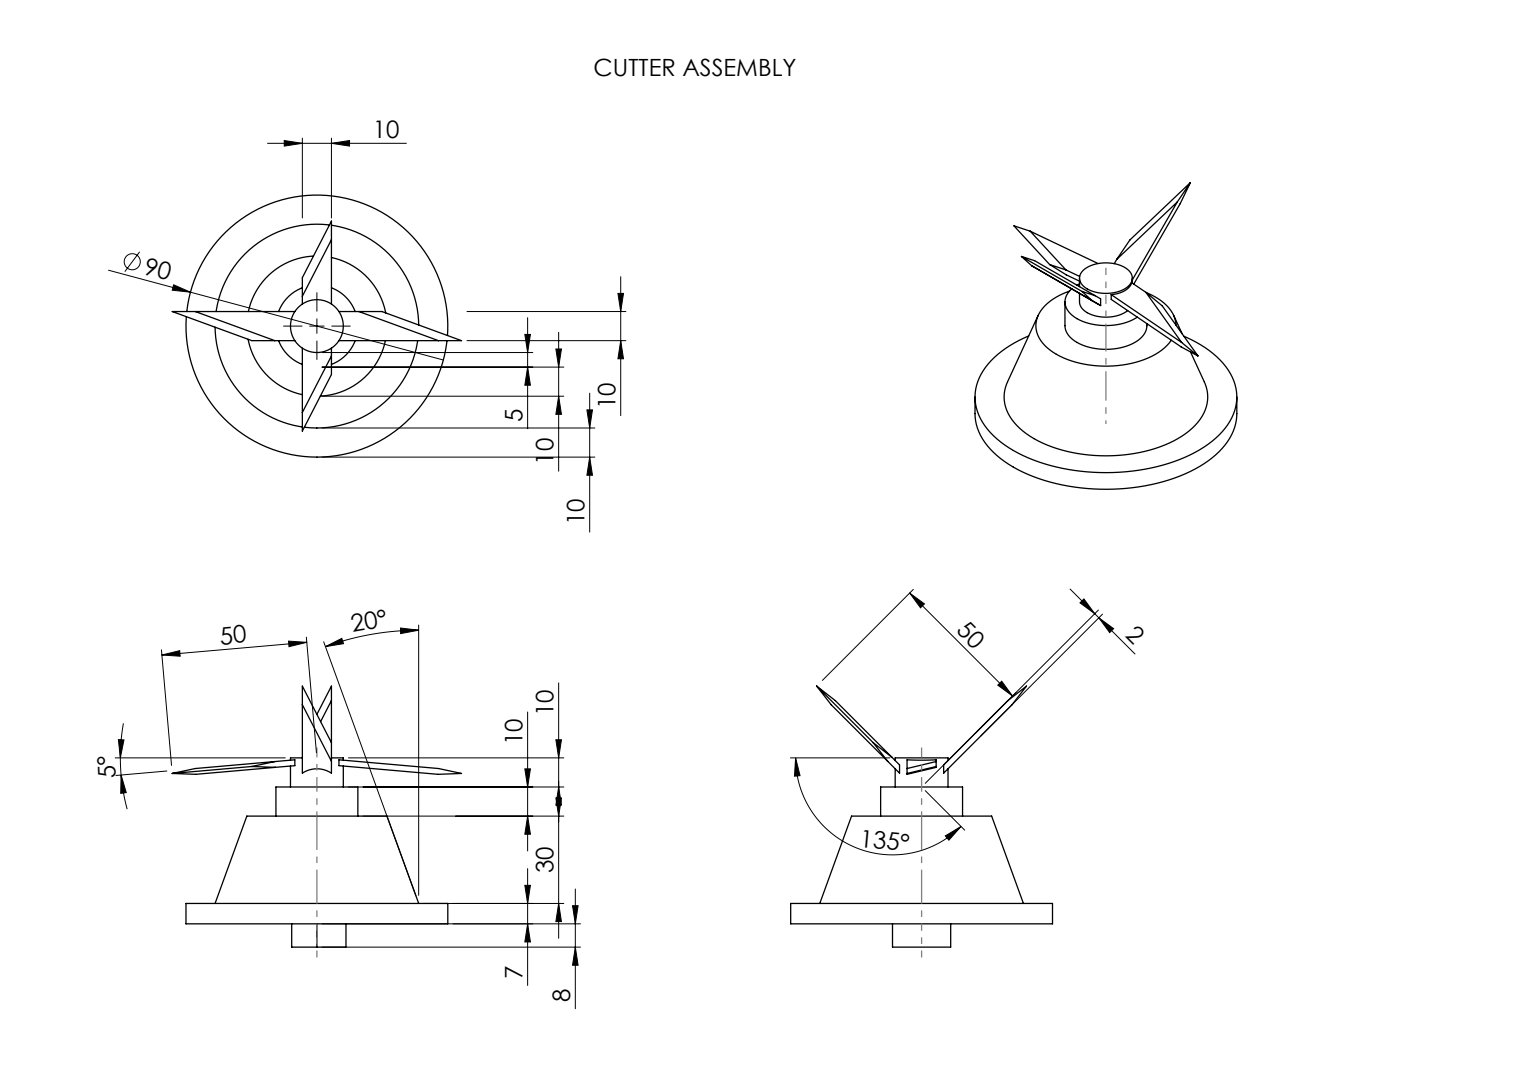
ISO-10303-21;
HEADER;
FILE_DESCRIPTION (('STEP AP214'),
    '1' );
FILE_NAME ('cutter assembly.step',
    '2026-10-09T15:02:13',
    ( '' ),
    ( '' ),
    'SwSTEP 2.0',
    'SolidWorks 2026',
    '' );
FILE_SCHEMA (( 'AUTOMOTIVE_DESIGN' ));
ENDSEC;

DATA;
#1=EDGE_CURVE ( 'NONE', #9758, #2312, #3659, .T. ) ;
#30=LINE ( 'NONE', #10110, #8655 ) ;
#58=VERTEX_POINT ( 'NONE', #12787 ) ;
#66=CARTESIAN_POINT ( 'NONE',  ( 9.262651381018932677E-15, 92.00000000000001421, -9.080892972013931086 ) ) ;
#71=ADVANCED_FACE ( 'NONE', ( #2644 ), #15361, .T. ) ;
#93=AXIS2_PLACEMENT_3D ( 'NONE', #810, #7225, #14526 ) ;
#117=CARTESIAN_POINT ( 'NONE',  ( -3.505380114644273348, 97.73782665365220623, 8.566253778398339236 ) ) ;
#119=ORIENTED_EDGE ( 'NONE', *, *, #8529, .T. ) ;
#143=CARTESIAN_POINT ( 'NONE',  ( 5.000000000000000000, 90.58578643762692195, -1.414213562373097588 ) ) ;
#172=VERTEX_POINT ( 'NONE', #11782 ) ;
#182=CARTESIAN_POINT ( 'NONE',  ( 9.227956911499398113E-15, 102.0000000000000142, -9.080892972013931086 ) ) ;
#202=CARTESIAN_POINT ( 'NONE',  ( 5.000000000000000000, 96.75198296766784267, -7.580410092414001433 ) ) ;
#213=EDGE_CURVE ( 'NONE', #982, #10751, #1081, .T. ) ;
#214=DIRECTION ( 'NONE',  ( 6.938893903907231459E-18, -1.000000000000000000, -5.551115123125782702E-17 ) ) ;
#218=PLANE ( 'NONE',  #7160 ) ;
#231=CARTESIAN_POINT ( 'NONE',  ( -49.72257916183962578, 96.64601816452537264, -5.000000000000008882 ) ) ;
#235=CARTESIAN_POINT ( 'NONE',  ( 9.332040320058006538E-15, 82.00000000000001421, -14.08089297201393286 ) ) ;
#296=DIRECTION ( 'NONE',  ( 0.000000000000000000, -0.7071067811865487940, -0.7071067811865463515 ) ) ;
#306=VERTEX_POINT ( 'NONE', #6172 ) ;
#321=CARTESIAN_POINT ( 'NONE',  ( -0.1743114854953159432, 100.0076106038165165, -5.000000000000000000 ) ) ;
#332=VERTEX_POINT ( 'NONE', #9993 ) ;
#335=DIRECTION ( 'NONE',  ( -5.069245582283711292E-17, -1.000000000000000000, 8.780190904559502465E-17 ) ) ;
#357=CARTESIAN_POINT ( 'NONE',  ( 5.000000000000000000, 102.0000000000000142, -7.580410092414002321 ) ) ;
#401=COLOUR_RGB ( '', 0.72549020, 0.75294118, 0.79215686) ;
#416=DIRECTION ( 'NONE',  ( -0.3420201433256697121, -0.6644630243886754384, 0.6644630243886734400 ) ) ;
#431=VECTOR ( 'NONE', #921, 1000.000000000000114 ) ;
#437=CARTESIAN_POINT ( 'NONE',  ( 9.234334497652928468E-15, 101.0808929720139702, -9.080892972013931086 ) ) ;
#456=CARTESIAN_POINT ( 'NONE',  ( -7.580410092413954359, 101.3368000520362813, 5.000000000000000000 ) ) ;
#457=CARTESIAN_POINT ( 'NONE',  ( 9.574901606694759531E-15, 52.00000000000001421, -2.191293403013901479E-14 ) ) ;
#460=ADVANCED_FACE ( 'NONE', ( #10847 ), #14901, .F. ) ;
#467=ORIENTED_EDGE ( 'NONE', *, *, #5813, .T. ) ;
#473=CARTESIAN_POINT ( 'NONE',  ( 5.000000000000000000, 92.00000000000001421, 0.000000000000000000 ) ) ;
#477=DIRECTION ( 'NONE',  ( 0.9361168066628590134, -0.08189960831908912886, 0.3420201433256691570 ) ) ;
#481=FILL_AREA_STYLE_COLOUR ( '', #401 ) ;
#487=ORIENTED_EDGE ( 'NONE', *, *, #6442, .T. ) ;
#492=AXIS2_PLACEMENT_3D ( 'NONE', #10068, #2407, #11397 ) ;
#499=FACE_OUTER_BOUND ( 'NONE', #6302, .T. ) ;
#506=ADVANCED_FACE ( 'NONE', ( #2101 ), #15988, .T. ) ;
#507=FACE_OUTER_BOUND ( 'NONE', #6954, .T. ) ;
#529=ADVANCED_FACE ( 'NONE', ( #2178 ), #12250, .T. ) ;
#536=DIRECTION ( 'NONE',  ( 0.000000000000000000, -1.541976423090494894E-16, -1.000000000000000000 ) ) ;
#537=DIRECTION ( 'NONE',  ( -0.000000000000000000, -0.6143407043256620126, -0.7890408728378077718 ) ) ;
#545=ORIENTED_EDGE ( 'NONE', *, *, #14628, .F. ) ;
#548=ORIENTED_EDGE ( 'NONE', *, *, #4265, .T. ) ;
#558=CARTESIAN_POINT ( 'NONE',  ( 1.875620865444973696E-15, 37.00000000000001421, -3.248670634687016947E-15 ) ) ;
#600=AXIS2_PLACEMENT_3D ( 'NONE', #14454, #6924, #1670 ) ;
#606=EDGE_CURVE ( 'NONE', #16014, #2610, #15398, .T. ) ;
#622=EDGE_LOOP ( 'NONE', ( #7600, #10634, #1804, #893 ) ) ;
#624=ORIENTED_EDGE ( 'NONE', *, *, #14015, .F. ) ;
#642=( GEOMETRIC_REPRESENTATION_CONTEXT ( 3 ) GLOBAL_UNCERTAINTY_ASSIGNED_CONTEXT ( ( #2937 ) ) GLOBAL_UNIT_ASSIGNED_CONTEXT ( ( #15209, #12566, #3759 ) ) REPRESENTATION_CONTEXT ( 'NONE', 'WORKASPACE' ) );
#648=DIRECTION ( 'NONE',  ( 0.000000000000000000, 8.780190904559502465E-17, 1.000000000000000000 ) ) ;
#650=ORIENTED_EDGE ( 'NONE', *, *, #1309, .F. ) ;
#660=DIRECTION ( 'NONE',  ( 0.000000000000000000, 0.000000000000000000, 1.000000000000000000 ) ) ;
#664=DIRECTION ( 'NONE',  ( -0.9961946980917455452, 0.08715574274765797158, 0.000000000000000000 ) ) ;
#668=AXIS2_PLACEMENT_3D ( 'NONE', #6556, #5317, #14175 ) ;
#677=VECTOR ( 'NONE', #999, 1000.000000000000114 ) ;
#686=CARTESIAN_POINT ( 'NONE',  ( 5.000000000000000000, 92.00000000000001421, 0.000000000000000000 ) ) ;
#698=AXIS2_PLACEMENT_3D ( 'NONE', #9570, #3238, #12296 ) ;
#700=ORIENTED_EDGE ( 'NONE', *, *, #4864, .F. ) ;
#706=VECTOR ( 'NONE', #3589, 1000.000000000000114 ) ;
#733=CIRCLE ( 'NONE', #6335, 9.080892972013911546 ) ;
#757=VECTOR ( 'NONE', #2822, 1000.000000000000000 ) ;
#759=DIRECTION ( 'NONE',  ( 0.9361168066628589024, 0.08189960831908940642, 0.3420201433256691570 ) ) ;
#784=CARTESIAN_POINT ( 'NONE',  ( 9.642970592016636644, 101.1563493904846780, 1.872989114519530984 ) ) ;
#798=VERTEX_POINT ( 'NONE', #9337 ) ;
#810=CARTESIAN_POINT ( 'NONE',  ( 9.297345850538470396E-15, 92.00000000000001421, -1.969248798088869855E-14 ) ) ;
#815=EDGE_CURVE ( 'NONE', #11124, #14188, #16130, .T. ) ;
#840=ORIENTED_EDGE ( 'NONE', *, *, #2746, .T. ) ;
#853=DIRECTION ( 'NONE',  ( 0.000000000000000000, 0.7071067811865487940, 0.7071067811865463515 ) ) ;
#877=ORIENTED_EDGE ( 'NONE', *, *, #7745, .T. ) ;
#893=ORIENTED_EDGE ( 'NONE', *, *, #4265, .F. ) ;
#894=VERTEX_POINT ( 'NONE', #14312 ) ;
#899=DIRECTION ( 'NONE',  ( -1.000000000000000000, 0.000000000000000000, -0.000000000000000000 ) ) ;
#907=ADVANCED_FACE ( 'NONE', ( #507 ), #6097, .T. ) ;
#916=ADVANCED_FACE ( 'NONE', ( #11164 ), #4772, .F. ) ;
#921=DIRECTION ( 'NONE',  ( 0.9361168066628589024, 0.08189960831908940642, 0.3420201433256691015 ) ) ;
#948=CARTESIAN_POINT ( 'NONE',  ( 7.580410092413973011, 101.3368000520362813, 5.000000000000000000 ) ) ;
#953=AXIS2_PLACEMENT_3D ( 'NONE', #5436, #10499, #15557 ) ;
#962=ORIENTED_EDGE ( 'NONE', *, *, #15661, .F. ) ;
#965=CARTESIAN_POINT ( 'NONE',  ( 9.297345850538470396E-15, 92.00000000000001421, -1.969248798088869855E-14 ) ) ;
#982=VERTEX_POINT ( 'NONE', #15894 ) ;
#991=DIRECTION ( 'NONE',  ( -0.9961946980917455452, -0.08715574274765824914, 0.000000000000000000 ) ) ;
#999=DIRECTION ( 'NONE',  ( 0.9961946980917455452, 0.08715574274765823526, -0.000000000000000000 ) ) ;
#1008=DIRECTION ( 'NONE',  ( 0.000000000000000000, -5.551115123125782702E-17, 1.000000000000000000 ) ) ;
#1023=ORIENTED_EDGE ( 'NONE', *, *, #9637, .F. ) ;
#1026=EDGE_LOOP ( 'NONE', ( #3436, #11766, #12269, #6841, #5637 ) ) ;
#1031=FACE_OUTER_BOUND ( 'NONE', #11108, .T. ) ;
#1049=EDGE_CURVE ( 'NONE', #3882, #11932, #14795, .T. ) ;
#1065=CARTESIAN_POINT ( 'NONE',  ( 0.000000000000000000, 0.000000000000000000, 5.000000000000000000 ) ) ;
#1071=CARTESIAN_POINT ( 'NONE',  ( -4.999999999999995559, 126.6482322781408953, 36.06244584051386681 ) ) ;
#1081=LINE ( 'NONE', #7492, #677 ) ;
#1103=ORIENTED_EDGE ( 'NONE', *, *, #11803, .F. ) ;
#1120=EDGE_CURVE ( 'NONE', #12156, #9153, #4935, .T. ) ;
#1143=DIRECTION ( 'NONE',  ( 0.000000000000000000, -0.7071067811865487940, 0.7071067811865463515 ) ) ;
#1144=AXIS2_PLACEMENT_3D ( 'NONE', #13530, #1964, #3307 ) ;
#1163=DIRECTION ( 'NONE',  ( 0.000000000000000000, 0.000000000000000000, 1.000000000000000000 ) ) ;
#1199=CARTESIAN_POINT ( 'NONE',  ( -5.000000000000000000, 96.75198296766780004, 7.580410092413951695 ) ) ;
#1204=VECTOR ( 'NONE', #296, 1000.000000000000000 ) ;
#1206=ORIENTED_EDGE ( 'NONE', *, *, #5813, .F. ) ;
#1213=CARTESIAN_POINT ( 'NONE',  ( 5.000000000000000000, 121.6750890729884134, -29.67508907298829968 ) ) ;
#1225=ORIENTED_EDGE ( 'NONE', *, *, #15661, .T. ) ;
#1232=DIRECTION ( 'NONE',  ( -0.000000000000000000, 0.7071067811865463515, 0.7071067811865487940 ) ) ;
#1281=CYLINDRICAL_SURFACE ( 'NONE', #5229, 45.00000000000000711 ) ;
#1304=DIRECTION ( 'NONE',  ( 0.000000000000000000, 0.000000000000000000, 1.000000000000000000 ) ) ;
#1309=EDGE_CURVE ( 'NONE', #16149, #10856, #13257, .T. ) ;
#1330=PRESENTATION_STYLE_ASSIGNMENT (( #6175 ) ) ;
#1350=ORIENTED_EDGE ( 'NONE', *, *, #10278, .F. ) ;
#1375=CARTESIAN_POINT ( 'NONE',  ( -22.35235477796478420, 99.04060251627524281, 5.000000000000000000 ) ) ;
#1387=VECTOR ( 'NONE', #16201, 1000.000000000000000 ) ;
#1407=VERTEX_POINT ( 'NONE', #4654 ) ;
#1422=CARTESIAN_POINT ( 'NONE',  ( 1.034004556265705202E-14, 102.0000000000000142, 9.080892972013893782 ) ) ;
#1444=CARTESIAN_POINT ( 'NONE',  ( 9.574901606694759531E-15, 52.00000000000001421, -2.191293403013901479E-14 ) ) ;
#1459=LINE ( 'NONE', #13398, #6549 ) ;
#1460=DIRECTION ( 'NONE',  ( 0.000000000000000000, 0.7071067811865487940, -0.7071067811865463515 ) ) ;
#1567=DIRECTION ( 'NONE',  ( -0.000000000000000000, 0.7071067811865463515, 0.7071067811865487940 ) ) ;
#1575=( LENGTH_UNIT ( ) NAMED_UNIT ( * ) SI_UNIT ( .MILLI., .METRE. ) );
#1602=VERTEX_POINT ( 'NONE', #202 ) ;
#1644=CARTESIAN_POINT ( 'NONE',  ( 22.35235477796478420, 99.04060251627522860, -5.000000000000000000 ) ) ;
#1670=DIRECTION ( 'NONE',  ( -0.5000000000000042188, 0.000000000000000000, -0.8660254037844362651 ) ) ;
#1688=CARTESIAN_POINT ( 'NONE',  ( 5.849792707072439590, 106.0483007247212015, 5.000000000000000888 ) ) ;
#1690=AXIS2_PLACEMENT_3D ( 'NONE', #3485, #4748, #13609 ) ;
#1716=VERTEX_POINT ( 'NONE', #10648 ) ;
#1717=EDGE_CURVE ( 'NONE', #15230, #9017, #14369, .T. ) ;
#1733=DIRECTION ( 'NONE',  ( 6.520427397917948411E-18, -0.9396926207859082059, 0.3420201433256693790 ) ) ;
#1743=ORIENTED_EDGE ( 'NONE', *, *, #10491, .F. ) ;
#1745=FACE_OUTER_BOUND ( 'NONE', #7603, .T. ) ;
#1750=DIRECTION ( 'NONE',  ( 0.9961946980917455452, -0.08715574274765797158, 0.000000000000000000 ) ) ;
#1755=DIRECTION ( 'NONE',  ( -0.9961946980917455452, 0.08715574274765797158, 0.000000000000000000 ) ) ;
#1758=DIRECTION ( 'NONE',  ( -0.3213938048432631867, -0.7471788047720969717, 0.5817472440052561256 ) ) ;
#1786=VECTOR ( 'NONE', #13203, 999.9999999999998863 ) ;
#1802=ORIENTED_EDGE ( 'NONE', *, *, #7646, .F. ) ;
#1804=ORIENTED_EDGE ( 'NONE', *, *, #1, .F. ) ;
#1809=CARTESIAN_POINT ( 'NONE',  ( -5.000000000000000000, 120.2608755106155201, 31.08930263536160155 ) ) ;
#1813=CARTESIAN_POINT ( 'NONE',  ( -5.000000000000000000, 58.69043703438383375, 45.69588935894790183 ) ) ;
#1868=CARTESIAN_POINT ( 'NONE',  ( -3.505380114644271572, 97.73782665365224887, -8.566253778398380092 ) ) ;
#1879=VERTEX_POINT ( 'NONE', #11455 ) ;
#1888=CARTESIAN_POINT ( 'NONE',  ( 48.69930661242913317, 95.73172307475270770, 7.581784256837345914 ) ) ;
#1890=DIRECTION ( 'NONE',  ( 0.9961946980917455452, -0.08715574274765795770, 0.000000000000000000 ) ) ;
#1914=CARTESIAN_POINT ( 'NONE',  ( -8.660254037844415720, 45.00000000000001421, -4.999999999999952927 ) ) ;
#1915=ORIENTED_EDGE ( 'NONE', *, *, #6442, .F. ) ;
#1926=CARTESIAN_POINT ( 'NONE',  ( 2.281160512027670796E-15, 45.00000000000001421, -3.951085907051776750E-15 ) ) ;
#1937=ORIENTED_EDGE ( 'NONE', *, *, #14545, .T. ) ;
#1941=EDGE_LOOP ( 'NONE', ( #13863, #12708 ) ) ;
#1964=DIRECTION ( 'NONE',  ( 5.069245582283711292E-17, 1.000000000000000000, -8.780190904559502465E-17 ) ) ;
#1989=CARTESIAN_POINT ( 'NONE',  ( 0.1743114854953164983, 100.0076106038165165, 5.000000000000000000 ) ) ;
#1996=DIRECTION ( 'NONE',  ( -6.938893903907231459E-18, 1.000000000000000000, 5.551115123125782702E-17 ) ) ;
#2008=EDGE_CURVE ( 'NONE', #5355, #10616, #15181, .T. ) ;
#2025=ORIENTED_EDGE ( 'NONE', *, *, #13441, .T. ) ;
#2049=EDGE_CURVE ( 'NONE', #12110, #4234, #733, .T. ) ;
#2051=VERTEX_POINT ( 'NONE', #16020 ) ;
#2053=DIRECTION ( 'NONE',  ( 0.000000000000000000, 0.000000000000000000, -1.000000000000000000 ) ) ;
#2058=DIRECTION ( 'NONE',  ( 0.9961946980917455452, 0.08715574274765823526, -0.000000000000000000 ) ) ;
#2069=ADVANCED_FACE ( 'NONE', ( #3305 ), #9800, .T. ) ;
#2071=CARTESIAN_POINT ( 'NONE',  ( -5.000000000000000000, 126.6482322781408953, 36.06244584051386681 ) ) ;
#2075=CARTESIAN_POINT ( 'NONE',  ( 4.890515327186546912, 101.5721353500714059, -8.487905985326070990 ) ) ;
#2083=CARTESIAN_POINT ( 'NONE',  ( -0.1743114854953159432, 100.0076106038165165, 5.000000000000000000 ) ) ;
#2101=FACE_OUTER_BOUND ( 'NONE', #2518, .T. ) ;
#2127=CARTESIAN_POINT ( 'NONE',  ( -5.000000000000000000, 96.75198296766780004, 7.580410092413951695 ) ) ;
#2136=CARTESIAN_POINT ( 'NONE',  ( -9.642970592016617104, 101.1563493904846780, 1.872989114519528986 ) ) ;
#2137=FACE_BOUND ( 'NONE', #5513, .T. ) ;
#2158=CARTESIAN_POINT ( 'NONE',  ( 0.000000000000000000, 0.000000000000000000, 0.000000000000000000 ) ) ;
#2167=ORIENTED_EDGE ( 'NONE', *, *, #2746, .F. ) ;
#2178=FACE_OUTER_BOUND ( 'NONE', #5573, .T. ) ;
#2186=ORIENTED_EDGE ( 'NONE', *, *, #8364, .F. ) ;
#2190=DIRECTION ( 'NONE',  ( -5.069245582283711292E-17, -1.000000000000000000, 8.780190904559502465E-17 ) ) ;
#2215=CARTESIAN_POINT ( 'NONE',  ( 7.580410092413973011, 102.0000000000000142, 5.000000000000000000 ) ) ;
#2227=VECTOR ( 'NONE', #6565, 1000.000000000000114 ) ;
#2269=APPLICATION_CONTEXT ( 'automotive_design' ) ;
#2273=VERTEX_POINT ( 'NONE', #6220 ) ;
#2288=AXIS2_PLACEMENT_3D ( 'NONE', #1926, #4787, #14563 ) ;
#2289=AXIS2_PLACEMENT_3D ( 'NONE', #2983, #4908, #8616 ) ;
#2290=AXIS2_PLACEMENT_3D ( 'NONE', #12049, #5593, #648 ) ;
#2312=VERTEX_POINT ( 'NONE', #3727 ) ;
#2328=CARTESIAN_POINT ( 'NONE',  ( -5.000000000000000000, 90.58578643762692195, -1.414213562373097588 ) ) ;
#2331=EDGE_CURVE ( 'NONE', #10856, #10814, #2549, .T. ) ;
#2345=EDGE_CURVE ( 'NONE', #2458, #11124, #10403, .T. ) ;
#2364=AXIS2_PLACEMENT_3D ( 'NONE', #1989, #7085, #991 ) ;
#2384=CARTESIAN_POINT ( 'NONE',  ( 9.227956911499398113E-15, 102.0000000000000142, -1.913737646857611713E-14 ) ) ;
#2394=EDGE_CURVE ( 'NONE', #12657, #2563, #15354, .T. ) ;
#2400=CARTESIAN_POINT ( 'NONE',  ( -8.660254037844415720, 37.00000000000001421, -4.999999999999952038 ) ) ;
#2402=PLANE ( 'NONE',  #7030 ) ;
#2407=DIRECTION ( 'NONE',  ( 5.069245582283711292E-17, 1.000000000000000000, -8.780190904559503697E-17 ) ) ;
#2458=VERTEX_POINT ( 'NONE', #12480 ) ;
#2475=ORIENTED_EDGE ( 'NONE', *, *, #8085, .T. ) ;
#2478=ORIENTED_EDGE ( 'NONE', *, *, #3150, .T. ) ;
#2486=CARTESIAN_POINT ( 'NONE',  ( 3.505380114644276013, 97.73782665365222044, -8.566253778398381868 ) ) ;
#2489=ADVANCED_FACE ( 'NONE', ( #6091 ), #8318, .F. ) ;
#2497=ORIENTED_EDGE ( 'NONE', *, *, #7202, .T. ) ;
#2518=EDGE_LOOP ( 'NONE', ( #1350, #9486, #15705, #9836 ) ) ;
#2519=VECTOR ( 'NONE', #16394, 1000.000000000000000 ) ;
#2535=ADVANCED_FACE ( 'NONE', ( #14791, #8485 ), #5836, .T. ) ;
#2539=CARTESIAN_POINT ( 'NONE',  ( 3.505380114644273348, 100.5662537783983765, 8.566253778398346341 ) ) ;
#2543=VECTOR ( 'NONE', #8638, 1000.000000000000227 ) ;
#2549=LINE ( 'NONE', #6306, #10050 ) ;
#2560=ORIENTED_EDGE ( 'NONE', *, *, #12839, .T. ) ;
#2563=VERTEX_POINT ( 'NONE', #8728 ) ;
#2593=CARTESIAN_POINT ( 'NONE',  ( 5.853156874688941503E-15, 82.00000000000001421, -24.08089297201393109 ) ) ;
#2610=VERTEX_POINT ( 'NONE', #66 ) ;
#2639=LINE ( 'NONE', #5248, #7511 ) ;
#2641=ADVANCED_FACE ( 'NONE', ( #15122 ), #15043, .T. ) ;
#2644=FACE_OUTER_BOUND ( 'NONE', #11195, .T. ) ;
#2687=ORIENTED_EDGE ( 'NONE', *, *, #12513, .T. ) ;
#2711=CARTESIAN_POINT ( 'NONE',  ( 0.000000000000000000, 0.000000000000000000, -5.000000000000000000 ) ) ;
#2716=DIRECTION ( 'NONE',  ( 0.9961946980917455452, 0.08715574274765824914, 0.000000000000000000 ) ) ;
#2738=DIRECTION ( 'NONE',  ( -1.000000000000000000, 0.000000000000000000, -0.000000000000000000 ) ) ;
#2745=DIRECTION ( 'NONE',  ( 0.000000000000000000, 0.000000000000000000, 1.000000000000000000 ) ) ;
#2746=EDGE_CURVE ( 'NONE', #3704, #798, #10472, .T. ) ;
#2775=EDGE_CURVE ( 'NONE', #9017, #306, #15530, .T. ) ;
#2791=DIRECTION ( 'NONE',  ( 0.000000000000000000, 8.780190904559502465E-17, 1.000000000000000000 ) ) ;
#2822=DIRECTION ( 'NONE',  ( 0.000000000000000000, 0.6143407043256605693, -0.7890408728378088821 ) ) ;
#2823=VECTOR ( 'NONE', #5091, 1000.000000000000114 ) ;
#2825=FILL_AREA_STYLE ('',( #481 ) ) ;
#2842=EDGE_CURVE ( 'NONE', #2273, #10236, #11393, .T. ) ;
#2843=CARTESIAN_POINT ( 'NONE',  ( -4.999999999999930722, 107.2206331336082741, -16.63484669598130949 ) ) ;
#2846=AXIS2_PLACEMENT_3D ( 'NONE', #2083, #11076, #664 ) ;
#2877=ORIENTED_EDGE ( 'NONE', *, *, #2842, .F. ) ;
#2879=AXIS2_PLACEMENT_3D ( 'NONE', #14621, #11236, #5920 ) ;
#2928=PLANE ( 'NONE',  #15020 ) ;
#2937=UNCERTAINTY_MEASURE_WITH_UNIT (LENGTH_MEASURE( 1.000000000000000082E-05 ), #15209, 'distance_accuracy_value', 'NONE');
#2976=FACE_OUTER_BOUND ( 'NONE', #5313, .T. ) ;
#2983=CARTESIAN_POINT ( 'NONE',  ( 9.297345850538470396E-15, 92.00000000000001421, -1.969248798088869855E-14 ) ) ;
#2984=SURFACE_STYLE_USAGE ( .BOTH. , #15778 ) ;
#2985=LINE ( 'NONE', #8054, #7018 ) ;
#2999=EDGE_LOOP ( 'NONE', ( #1023, #2877, #14697, #16344 ) ) ;
#3030=EDGE_CURVE ( 'NONE', #16226, #12784, #14768, .T. ) ;
#3041=CARTESIAN_POINT ( 'NONE',  ( 9.227956911499398113E-15, 102.0000000000000142, -9.080892972013931086 ) ) ;
#3062=( LENGTH_UNIT ( ) NAMED_UNIT ( * ) SI_UNIT ( .MILLI., .METRE. ) );
#3078=DIRECTION ( 'NONE',  ( 5.069245582283711292E-17, 1.000000000000000000, -8.780190904559502465E-17 ) ) ;
#3081=ORIENTED_EDGE ( 'NONE', *, *, #9637, .T. ) ;
#3082=PRODUCT_DEFINITION_SHAPE ( 'NONE', 'NONE',  #5699 ) ;
#3120=VECTOR ( 'NONE', #3176, 1000.000000000000114 ) ;
#3150=EDGE_CURVE ( 'NONE', #4234, #12110, #14835, .T. ) ;
#3151=DIRECTION ( 'NONE',  ( 0.9961946980917455452, -0.08715574274765797158, 0.000000000000000000 ) ) ;
#3153=VERTEX_POINT ( 'NONE', #1213 ) ;
#3166=ORIENTED_EDGE ( 'NONE', *, *, #8349, .T. ) ;
#3176=DIRECTION ( 'NONE',  ( 0.000000000000000000, 0.7890408728378107694, 0.6143407043256581268 ) ) ;
#3196=ORIENTED_EDGE ( 'NONE', *, *, #10399, .F. ) ;
#3205=ADVANCED_FACE ( 'NONE', ( #10373 ), #218, .T. ) ;
#3230=ORIENTED_EDGE ( 'NONE', *, *, #16166, .T. ) ;
#3238=DIRECTION ( 'NONE',  ( 6.938893903907231459E-18, -1.000000000000000000, -5.551115123125782702E-17 ) ) ;
#3260=PLANE ( 'NONE',  #5986 ) ;
#3273=DIRECTION ( 'NONE',  ( 0.1984322509960792513, 0.9259215214979028552, -0.3213938048432757877 ) ) ;
#3281=ORIENTED_EDGE ( 'NONE', *, *, #7386, .F. ) ;
#3294=CARTESIAN_POINT ( 'NONE',  ( 1.034642314881058238E-14, 101.0808929720139417, 9.080892972013893782 ) ) ;
#3295=EDGE_LOOP ( 'NONE', ( #12567, #487, #8570, #11224, #650, #2687, #2497, #6321, #3385, #5557, #13862, #8997 ) ) ;
#3305=FACE_OUTER_BOUND ( 'NONE', #14373, .T. ) ;
#3307=DIRECTION ( 'NONE',  ( 0.000000000000000000, 1.541976423090494894E-16, 1.000000000000000000 ) ) ;
#3343=VECTOR ( 'NONE', #15215, 1000.000000000000227 ) ;
#3385=ORIENTED_EDGE ( 'NONE', *, *, #15871, .F. ) ;
#3394=FACE_OUTER_BOUND ( 'NONE', #8230, .T. ) ;
#3423=ADVANCED_FACE ( 'NONE', ( #8804 ), #11392, .F. ) ;
#3429=CARTESIAN_POINT ( 'NONE',  ( 9.227956911499398113E-15, 102.0000000000000142, -1.913737646857611713E-14 ) ) ;
#3436=ORIENTED_EDGE ( 'NONE', *, *, #11535, .T. ) ;
#3485=CARTESIAN_POINT ( 'NONE',  ( 9.227956911499398113E-15, 102.0000000000000142, -1.913737646857611713E-14 ) ) ;
#3502=LINE ( 'NONE', #5262, #8940 ) ;
#3515=EDGE_LOOP ( 'NONE', ( #13115, #3081, #8654, #8363 ) ) ;
#3528=CARTESIAN_POINT ( 'NONE',  ( 4.890515327186548689, 101.5721353500714059, -8.487905985326074543 ) ) ;
#3531=AXIS2_PLACEMENT_3D ( 'NONE', #12865, #12783, #1304 ) ;
#3536=ORIENTED_EDGE ( 'NONE', *, *, #8529, .F. ) ;
#3538=ORIENTED_EDGE ( 'NONE', *, *, #5207, .T. ) ;
#3589=DIRECTION ( 'NONE',  ( 0.9777979793268661846, -0.2095497831645198317, 0.000000000000000000 ) ) ;
#3596=FACE_OUTER_BOUND ( 'NONE', #7045, .T. ) ;
#3607=EDGE_CURVE ( 'NONE', #15466, #1879, #8976, .T. ) ;
#3617=( GEOMETRIC_REPRESENTATION_CONTEXT ( 3 ) GLOBAL_UNCERTAINTY_ASSIGNED_CONTEXT ( ( #7760 ) ) GLOBAL_UNIT_ASSIGNED_CONTEXT ( ( #3062, #11717, #11960 ) ) REPRESENTATION_CONTEXT ( 'NONE', 'WORKASPACE' ) );
#3621=VERTEX_POINT ( 'NONE', #7725 ) ;
#3659=LINE ( 'NONE', #8715, #5745 ) ;
#3666=DIRECTION ( 'NONE',  ( 0.3213938048432681271, -0.5817472440052512406, 0.7471788047720988590 ) ) ;
#3676=DIRECTION ( 'NONE',  ( 0.3420201433256698231, -0.6644630243886754384, -0.6644630243886734400 ) ) ;
#3704=VERTEX_POINT ( 'NONE', #12029 ) ;
#3710=DIRECTION ( 'NONE',  ( -0.9993309688977880523, -0.03657341386592528887, -0.000000000000000000 ) ) ;
#3722=ORIENTED_EDGE ( 'NONE', *, *, #14933, .F. ) ;
#3724=DIRECTION ( 'NONE',  ( 0.000000000000000000, 0.000000000000000000, 1.000000000000000000 ) ) ;
#3727=CARTESIAN_POINT ( 'NONE',  ( 5.000000000000000000, 102.2474899284555931, 10.24748992845553808 ) ) ;
#3751=CARTESIAN_POINT ( 'NONE',  ( 21.27467419401223125, 99.27155792573854853, -5.000000000000000000 ) ) ;
#3759=( NAMED_UNIT ( * ) SI_UNIT ( $, .STERADIAN. ) SOLID_ANGLE_UNIT ( ) );
#3801=EDGE_LOOP ( 'NONE', ( #14574, #8800, #6894, #1206 ) ) ;
#3812=CARTESIAN_POINT ( 'NONE',  ( 1.102175790126979847E-14, 92.00000000000001421, 14.08089297201389201 ) ) ;
#3838=ORIENTED_EDGE ( 'NONE', *, *, #3607, .T. ) ;
#3859=VECTOR ( 'NONE', #4778, 999.9999999999998863 ) ;
#3882=VERTEX_POINT ( 'NONE', #1809 ) ;
#3886=PLANE ( 'NONE',  #668 ) ;
#3891=VECTOR ( 'NONE', #11737, 1000.000000000000000 ) ;
#3903=ORIENTED_EDGE ( 'NONE', *, *, #15238, .F. ) ;
#3904=VERTEX_POINT ( 'NONE', #15939 ) ;
#3925=ORIENTED_EDGE ( 'NONE', *, *, #12330, .F. ) ;
#3941=( BOUNDED_CURVE ( )  B_SPLINE_CURVE ( 3, ( #14660, #9537, #1868, #14581 ),
 .UNSPECIFIED., .F., .F. ) 
 B_SPLINE_CURVE_WITH_KNOTS ( ( 4, 4 ),
 ( 3.141592653589793116, 3.724683441357939273 ),
 .UNSPECIFIED. ) 
 CURVE ( )  GEOMETRIC_REPRESENTATION_ITEM ( )  RATIONAL_B_SPLINE_CURVE ( ( 1.000000000000000000, 0.9718672150731668680, 0.9718672150731668680, 1.000000000000000000 ) ) 
 REPRESENTATION_ITEM ( '' )  );
#3958=ORIENTED_EDGE ( 'NONE', *, *, #8349, .F. ) ;
#3981=VERTEX_POINT ( 'NONE', #12362 ) ;
#3984=AXIS2_PLACEMENT_3D ( 'NONE', #10064, #11543, #6159 ) ;
#3990=LINE ( 'NONE', #15196, #2823 ) ;
#3999=DIRECTION ( 'NONE',  ( 0.000000000000000000, 0.000000000000000000, -1.000000000000000000 ) ) ;
#4004=CARTESIAN_POINT ( 'NONE',  ( 9.366734789577542680E-15, 82.00000000000001421, -2.024759949320127682E-14 ) ) ;
#4005=DIRECTION ( 'NONE',  ( -0.000000000000000000, 0.6143407043256620126, 0.7890408728378077718 ) ) ;
#4015=CARTESIAN_POINT ( 'NONE',  ( -1.790468199911976477, 101.0808929720139417, 9.080892972013895559 ) ) ;
#4043=ORIENTED_EDGE ( 'NONE', *, *, #5569, .T. ) ;
#4044=CARTESIAN_POINT ( 'NONE',  ( 41.80721665588484370, 98.34234248903790387, 5.000000000000000000 ) ) ;
#4045=FACE_OUTER_BOUND ( 'NONE', #1941, .T. ) ;
#4047=CARTESIAN_POINT ( 'NONE',  ( 1.790468199911984692, 101.0808929720139560, -9.080892972013931086 ) ) ;
#4079=ADVANCED_FACE ( 'NONE', ( #7788 ), #3886, .F. ) ;
#4086=EDGE_LOOP ( 'NONE', ( #6865, #14652, #10573, #14800, #6150 ) ) ;
#4133=ADVANCED_FACE ( 'NONE', ( #6467 ), #7626, .T. ) ;
#4149=ORIENTED_EDGE ( 'NONE', *, *, #12874, .T. ) ;
#4176=AXIS2_PLACEMENT_3D ( 'NONE', #14537, #3078, #15708 ) ;
#4186=FACE_OUTER_BOUND ( 'NONE', #3801, .T. ) ;
#4201=LINE ( 'NONE', #13245, #4420 ) ;
#4209=LINE ( 'NONE', #357, #7602 ) ;
#4220=DIRECTION ( 'NONE',  ( -5.069245582283711292E-17, -1.000000000000000000, 8.780190904559502465E-17 ) ) ;
#4228=AXIS2_PLACEMENT_3D ( 'NONE', #11641, #7975, #15450 ) ;
#4234=VERTEX_POINT ( 'NONE', #5390 ) ;
#4244=CARTESIAN_POINT ( 'NONE',  ( 1.036604930454412972E-14, 98.25246584726775723, 9.080892972013893782 ) ) ;
#4246=FACE_BOUND ( 'NONE', #10138, .T. ) ;
#4265=EDGE_CURVE ( 'NONE', #11932, #9758, #8276, .T. ) ;
#4269=CARTESIAN_POINT ( 'NONE',  ( 4.350898428888834396E-14, 37.00000000000001421, 10.00000000000000355 ) ) ;
#4300=DIRECTION ( 'NONE',  ( 5.069245582283711292E-17, 1.000000000000000000, -8.780190904559502465E-17 ) ) ;
#4310=EDGE_LOOP ( 'NONE', ( #14073, #7050, #15037, #14295 ) ) ;
#4317=EDGE_CURVE ( 'NONE', #13593, #2563, #14910, .T. ) ;
#4330=ORIENTED_EDGE ( 'NONE', *, *, #6165, .T. ) ;
#4343=CARTESIAN_POINT ( 'NONE',  ( 5.000000000000000000, 120.2608755106154348, -31.08930263536150562 ) ) ;
#4403=PRESENTATION_STYLE_ASSIGNMENT (( #2984 ) ) ;
#4406=AXIS2_PLACEMENT_3D ( 'NONE', #5389, #4300, #2791 ) ;
#4420=VECTOR ( 'NONE', #5683, 1000.000000000000114 ) ;
#4486=DIRECTION ( 'NONE',  ( 0.000000000000000000, 0.000000000000000000, 1.000000000000000000 ) ) ;
#4492=LINE ( 'NONE', #2215, #11519 ) ;
#4497=ADVANCED_FACE ( 'NONE', ( #12841 ), #1281, .T. ) ;
#4500=ORIENTED_EDGE ( 'NONE', *, *, #10739, .F. ) ;
#4503=AXIS2_PLACEMENT_3D ( 'NONE', #13711, #10901, #7411 ) ;
#4514=PLANE ( 'NONE',  #6474 ) ;
#4528=EDGE_CURVE ( 'NONE', #894, #15230, #9100, .T. ) ;
#4542=ORIENTED_EDGE ( 'NONE', *, *, #2775, .F. ) ;
#4560=CARTESIAN_POINT ( 'NONE',  ( 5.000000000000000000, 90.81335289333328831, 3.860273862222790342 ) ) ;
#4579=PLANE ( 'NONE',  #9956 ) ;
#4584=CARTESIAN_POINT ( 'NONE',  ( 49.72257916183961868, 96.64601816452534422, 5.000000000000000000 ) ) ;
#4621=EDGE_LOOP ( 'NONE', ( #840, #11868, #5108, #8104, #5406 ) ) ;
#4629=PLANE ( 'NONE',  #9706 ) ;
#4641=EDGE_CURVE ( 'NONE', #798, #15902, #30, .T. ) ;
#4654=CARTESIAN_POINT ( 'NONE',  ( 5.288637809679021457E-15, 52.00000000000001421, -35.00000000000002842 ) ) ;
#4657=ORIENTED_EDGE ( 'NONE', *, *, #14015, .T. ) ;
#4658=CIRCLE ( 'NONE', #13660, 35.00000000000000711 ) ;
#4676=( GEOMETRIC_REPRESENTATION_CONTEXT ( 3 ) GLOBAL_UNCERTAINTY_ASSIGNED_CONTEXT ( ( #10912 ) ) GLOBAL_UNIT_ASSIGNED_CONTEXT ( ( #1575, #5503, #9475 ) ) REPRESENTATION_CONTEXT ( 'NONE', 'WORKASPACE' ) );
#4679=( BOUNDED_CURVE ( )  B_SPLINE_CURVE ( 3, ( #1199, #117, #15251, #8864 ),
 .UNSPECIFIED., .F., .F. ) 
 B_SPLINE_CURVE_WITH_KNOTS ( ( 4, 4 ),
 ( 2.558501865821646959, 3.141592653589793116 ),
 .UNSPECIFIED. ) 
 CURVE ( )  GEOMETRIC_REPRESENTATION_ITEM ( )  RATIONAL_B_SPLINE_CURVE ( ( 1.000000000000000000, 0.9718672150731668680, 0.9718672150731668680, 1.000000000000000000 ) ) 
 REPRESENTATION_ITEM ( '' )  );
#4688=VECTOR ( 'NONE', #11977, 1000.000000000000114 ) ;
#4690=ORIENTED_EDGE ( 'NONE', *, *, #8627, .F. ) ;
#4697=DIRECTION ( 'NONE',  ( 0.000000000000000000, 0.000000000000000000, 1.000000000000000000 ) ) ;
#4713=EDGE_CURVE ( 'NONE', #9419, #3904, #15566, .T. ) ;
#4737=EDGE_LOOP ( 'NONE', ( #5049, #16013, #12238, #8926 ) ) ;
#4748=DIRECTION ( 'NONE',  ( 6.938893903907231459E-18, -1.000000000000000000, -5.551115123125782702E-17 ) ) ;
#4759=FACE_OUTER_BOUND ( 'NONE', #13729, .T. ) ;
#4762=FACE_OUTER_BOUND ( 'NONE', #12008, .T. ) ;
#4772=PLANE ( 'NONE',  #2846 ) ;
#4777=ORIENTED_EDGE ( 'NONE', *, *, #2394, .F. ) ;
#4778=DIRECTION ( 'NONE',  ( 0.000000000000000000, 0.7071067811865487940, -0.7071067811865463515 ) ) ;
#4779=EDGE_LOOP ( 'NONE', ( #11743, #16056, #16210, #15253, #5887 ) ) ;
#4787=DIRECTION ( 'NONE',  ( -5.069245582283711292E-17, -1.000000000000000000, 8.780190904559502465E-17 ) ) ;
#4861=ORIENTED_EDGE ( 'NONE', *, *, #815, .F. ) ;
#4864=EDGE_CURVE ( 'NONE', #10616, #16078, #5746, .T. ) ;
#4908=DIRECTION ( 'NONE',  ( -6.938893903907231459E-18, 1.000000000000000000, 5.551115123125782702E-17 ) ) ;
#4913=LINE ( 'NONE', #5079, #1387 ) ;
#4935=LINE ( 'NONE', #3751, #706 ) ;
#4944=DIRECTION ( 'NONE',  ( -1.000000000000000000, 0.000000000000000000, 0.000000000000000000 ) ) ;
#4958=AXIS2_PLACEMENT_3D ( 'NONE', #10367, #214, #12857 ) ;
#4967=CLOSED_SHELL ( 'NONE', ( #4133, #11945, #9888, #2535, #9968, #7240, #4497, #11822, #12516, #9974, #9380, #13799, #907, #14274, #71, #2489, #5802, #5210, #8839, #3205, #916, #8610, #11903, #506, #4079, #16402, #11304, #8143, #529, #3423, #12587, #8990, #9356, #2069, #460, #14023, #8211, #2641, #15494, #7086 ) ) ;
#4978=LINE ( 'NONE', #6133, #6463 ) ;
#5021=EDGE_CURVE ( 'NONE', #5355, #172, #13702, .T. ) ;
#5049=ORIENTED_EDGE ( 'NONE', *, *, #16166, .F. ) ;
#5059=CARTESIAN_POINT ( 'NONE',  ( 7.580410092413998768, 102.0000000000000142, -5.000000000000000000 ) ) ;
#5079=CARTESIAN_POINT ( 'NONE',  ( 5.000000000000000888, 99.08339874278649972, -0.6589959970937100397 ) ) ;
#5084=ORIENTED_EDGE ( 'NONE', *, *, #5207, .F. ) ;
#5091=DIRECTION ( 'NONE',  ( -0.5000000000000042188, -0.000000000000000000, -0.8660254037844362651 ) ) ;
#5100=ORIENTED_EDGE ( 'NONE', *, *, #4713, .T. ) ;
#5108=ORIENTED_EDGE ( 'NONE', *, *, #5330, .F. ) ;
#5144=VECTOR ( 'NONE', #10660, 1000.000000000000114 ) ;
#5163=ORIENTED_EDGE ( 'NONE', *, *, #3030, .T. ) ;
#5205=ORIENTED_EDGE ( 'NONE', *, *, #9291, .T. ) ;
#5207=EDGE_CURVE ( 'NONE', #16078, #10616, #14229, .T. ) ;
#5210=ADVANCED_FACE ( 'NONE', ( #4186 ), #2928, .T. ) ;
#5211=CARTESIAN_POINT ( 'NONE',  ( -3.589930709342005422, 98.09116937221706678, -5.000000000000000000 ) ) ;
#5229=AXIS2_PLACEMENT_3D ( 'NONE', #1444, #10350, #7692 ) ;
#5244=LINE ( 'NONE', #15606, #2227 ) ;
#5248=CARTESIAN_POINT ( 'NONE',  ( 0.1743114854953164983, 100.0076106038165165, -5.000000000000000000 ) ) ;
#5262=CARTESIAN_POINT ( 'NONE',  ( -1.572311786628345809, 98.28009660169102801, 5.000000000000000000 ) ) ;
#5279=LINE ( 'NONE', #11566, #16085 ) ;
#5284=CARTESIAN_POINT ( 'NONE',  ( -3.505380114644273348, 100.5662537783983908, 8.566253778398339236 ) ) ;
#5313=EDGE_LOOP ( 'NONE', ( #119, #2025, #14356, #4861, #13040 ) ) ;
#5317=DIRECTION ( 'NONE',  ( -0.03463303435789753804, 0.9463120918278141724, 0.3213938048432660732 ) ) ;
#5320=DIRECTION ( 'NONE',  ( 0.000000000000000000, 0.7071067811865487940, -0.7071067811865463515 ) ) ;
#5321=DIRECTION ( 'NONE',  ( 0.000000000000000000, 0.000000000000000000, -1.000000000000000000 ) ) ;
#5328=DIRECTION ( 'NONE',  ( 0.9993309688977880523, 0.03657341386592528887, -0.000000000000000000 ) ) ;
#5330=EDGE_CURVE ( 'NONE', #3621, #15902, #12950, .T. ) ;
#5334=ORIENTED_EDGE ( 'NONE', *, *, #8123, .T. ) ;
#5355=VERTEX_POINT ( 'NONE', #10070 ) ;
#5359=PLANE ( 'NONE',  #600 ) ;
#5381=CARTESIAN_POINT ( 'NONE',  ( 1.490838860747792127E-14, 52.00000000000002132, 44.99999999999998579 ) ) ;
#5389=CARTESIAN_POINT ( 'NONE',  ( 9.220054415934899174E-15, 45.00000000000001421, -2.129832066681984848E-14 ) ) ;
#5390=CARTESIAN_POINT ( 'NONE',  ( 1.037474003217658816E-14, 102.0000000000000142, 9.080892972013893782 ) ) ;
#5406=ORIENTED_EDGE ( 'NONE', *, *, #9936, .T. ) ;
#5434=DIRECTION ( 'NONE',  ( 0.000000000000000000, 0.000000000000000000, 1.000000000000000000 ) ) ;
#5436=CARTESIAN_POINT ( 'NONE',  ( 9.366734789577542680E-15, 82.00000000000001421, -2.024759949320127682E-14 ) ) ;
#5448=ORIENTED_EDGE ( 'NONE', *, *, #11297, .T. ) ;
#5457=DIRECTION ( 'NONE',  ( 0.9777979793268667397, 0.2095497831645171394, -0.000000000000000000 ) ) ;
#5489=EDGE_CURVE ( 'NONE', #3882, #12433, #11316, .T. ) ;
#5503=( NAMED_UNIT ( * ) PLANE_ANGLE_UNIT ( ) SI_UNIT ( $, .RADIAN. ) );
#5510=ORIENTED_EDGE ( 'NONE', *, *, #6123, .T. ) ;
#5513=EDGE_LOOP ( 'NONE', ( #1743, #16277, #14277, #4657 ) ) ;
#5525=AXIS2_PLACEMENT_3D ( 'NONE', #3429, #1996, #13555 ) ;
#5547=CARTESIAN_POINT ( 'NONE',  ( 5.000000000000000000, 90.58578643762692195, -1.414213562373097588 ) ) ;
#5557=ORIENTED_EDGE ( 'NONE', *, *, #6127, .F. ) ;
#5569=EDGE_CURVE ( 'NONE', #12110, #11124, #15754, .T. ) ;
#5573=EDGE_LOOP ( 'NONE', ( #3925, #13135, #6838, #2186, #11428 ) ) ;
#5574=ORIENTED_EDGE ( 'NONE', *, *, #5489, .T. ) ;
#5593=DIRECTION ( 'NONE',  ( 5.069245582283711292E-17, 1.000000000000000000, -8.780190904559502465E-17 ) ) ;
#5600=CARTESIAN_POINT ( 'NONE',  ( -14.26268078651477822, 98.74453744460426208, 5.000000000000000000 ) ) ;
#5610=ORIENTED_EDGE ( 'NONE', *, *, #8539, .F. ) ;
#5622=EDGE_CURVE ( 'NONE', #16014, #3621, #3941, .T. ) ;
#5629=ORIENTED_EDGE ( 'NONE', *, *, #13441, .F. ) ;
#5637=ORIENTED_EDGE ( 'NONE', *, *, #14308, .F. ) ;
#5641=( BOUNDED_CURVE ( )  B_SPLINE_CURVE ( 3, ( #11492, #5284, #4015, #6186 ),
 .UNSPECIFIED., .F., .T. ) 
 B_SPLINE_CURVE_WITH_KNOTS ( ( 4, 4 ),
 ( 2.558501865821646959, 3.141592653589793116 ),
 .UNSPECIFIED. ) 
 CURVE ( )  GEOMETRIC_REPRESENTATION_ITEM ( )  RATIONAL_B_SPLINE_CURVE ( ( 1.000000000000000000, 0.9718672150731668680, 0.9718672150731668680, 1.000000000000000000 ) ) 
 REPRESENTATION_ITEM ( '' )  );
#5656=CARTESIAN_POINT ( 'NONE',  ( 5.000000000000000000, 92.00000000000001421, 0.000000000000000000 ) ) ;
#5660=ORIENTED_EDGE ( 'NONE', *, *, #4641, .F. ) ;
#5668=LINE ( 'NONE', #10735, #13955 ) ;
#5669=LINE ( 'NONE', #2843, #5144 ) ;
#5675=CARTESIAN_POINT ( 'NONE',  ( 9.234334497652928468E-15, 101.0808929720139702, -9.080892972013931086 ) ) ;
#5683=DIRECTION ( 'NONE',  ( -0.3420201433256697121, 0.6644630243886755494, 0.6644630243886733290 ) ) ;
#5699=PRODUCT_DEFINITION ( 'UNKNOWN', '', #16346, #8415 ) ;
#5745=VECTOR ( 'NONE', #13780, 1000.000000000000114 ) ;
#5746=CIRCLE ( 'NONE', #14752, 14.08089297201391155 ) ;
#5747=VECTOR ( 'NONE', #416, 1000.000000000000114 ) ;
#5761=CARTESIAN_POINT ( 'NONE',  ( -5.000000000000000000, 30.31797207441543307, -38.93949884783829418 ) ) ;
#5802=ADVANCED_FACE ( 'NONE', ( #1031 ), #4629, .T. ) ;
#5813=EDGE_CURVE ( 'NONE', #58, #894, #7529, .T. ) ;
#5828=CARTESIAN_POINT ( 'NONE',  ( -1.514495797847258629, 99.85985911164404172, 9.657683769731226775 ) ) ;
#5836=CYLINDRICAL_SURFACE ( 'NONE', #4503, 9.080892972013911546 ) ;
#5861=DIRECTION ( 'NONE',  ( 0.000000000000000000, 0.7071067811865463515, -0.7071067811865487940 ) ) ;
#5887=ORIENTED_EDGE ( 'NONE', *, *, #3030, .F. ) ;
#5904=ORIENTED_EDGE ( 'NONE', *, *, #10739, .T. ) ;
#5911=DIRECTION ( 'NONE',  ( -0.03463303435789952950, -0.9463120918278121740, 0.3213938048432717909 ) ) ;
#5914=DIRECTION ( 'NONE',  ( 0.000000000000000000, 0.000000000000000000, 1.000000000000000000 ) ) ;
#5920=DIRECTION ( 'NONE',  ( 0.000000000000000000, 1.541976423090494894E-16, 1.000000000000000000 ) ) ;
#5940=DIRECTION ( 'NONE',  ( -6.938893903907231459E-18, 1.000000000000000000, 5.551115123125782702E-17 ) ) ;
#5951=VERTEX_POINT ( 'NONE', #5381 ) ;
#5953=ORIENTED_EDGE ( 'NONE', *, *, #7386, .T. ) ;
#5964=CIRCLE ( 'NONE', #9151, 14.08089297201391155 ) ;
#5981=( BOUNDED_CURVE ( )  B_SPLINE_CURVE ( 3, ( #8466, #11045, #2136, #7223 ),
 .UNSPECIFIED., .F., .F. ) 
 B_SPLINE_CURVE_WITH_KNOTS ( ( 4, 4 ),
 ( 5.700094519411444516, 6.866276094947734165 ),
 .UNSPECIFIED. ) 
 CURVE ( )  GEOMETRIC_REPRESENTATION_ITEM ( )  RATIONAL_B_SPLINE_CURVE ( ( 1.000000000000000000, 0.8898432210558864242, 0.8898432210558864242, 1.000000000000000000 ) ) 
 REPRESENTATION_ITEM ( '' )  );
#5986=AXIS2_PLACEMENT_3D ( 'NONE', #8330, #13394, #759 ) ;
#5994=FACE_OUTER_BOUND ( 'NONE', #3515, .T. ) ;
#6012=LINE ( 'NONE', #1914, #12828 ) ;
#6019=FACE_OUTER_BOUND ( 'NONE', #10672, .T. ) ;
#6036=ORIENTED_EDGE ( 'NONE', *, *, #7646, .T. ) ;
#6091=FACE_OUTER_BOUND ( 'NONE', #10889, .T. ) ;
#6097=PLANE ( 'NONE',  #5525 ) ;
#6123=EDGE_CURVE ( 'NONE', #1602, #15466, #9187, .T. ) ;
#6127=EDGE_CURVE ( 'NONE', #2458, #1602, #4209, .T. ) ;
#6129=CARTESIAN_POINT ( 'NONE',  ( 9.642970592016647302, 101.1563493904846780, -1.872989114519519882 ) ) ;
#6133=CARTESIAN_POINT ( 'NONE',  ( 7.581784256837408975, 125.2766624725656897, -36.10508959731173917 ) ) ;
#6150=ORIENTED_EDGE ( 'NONE', *, *, #5622, .T. ) ;
#6156=DIRECTION ( 'NONE',  ( 0.9361168066628589024, 0.08189960831908940642, 0.3420201433256691570 ) ) ;
#6158=DIRECTION ( 'NONE',  ( 0.000000000000000000, 0.7071067811865487940, 0.7071067811865463515 ) ) ;
#6159=DIRECTION ( 'NONE',  ( 0.000000000000000000, 0.000000000000000000, 1.000000000000000000 ) ) ;
#6165=EDGE_CURVE ( 'NONE', #1716, #982, #10609, .T. ) ;
#6172=CARTESIAN_POINT ( 'NONE',  ( 41.63290517038976901, 96.34995309285439191, 5.000000000000000000 ) ) ;
#6175=SURFACE_STYLE_USAGE ( .BOTH. , #15057 ) ;
#6177=CARTESIAN_POINT ( 'NONE',  ( -5.000000000000000000, 0.000000000000000000, 0.000000000000000000 ) ) ;
#6186=CARTESIAN_POINT ( 'NONE',  ( 1.034642314881058238E-14, 101.0808929720139417, 9.080892972013893782 ) ) ;
#6192=CIRCLE ( 'NONE', #3531, 35.00000000000000711 ) ;
#6220=CARTESIAN_POINT ( 'NONE',  ( 9.366734789577542680E-15, 82.00000000000001421, 24.08089297201388845 ) ) ;
#6284=AXIS2_PLACEMENT_3D ( 'NONE', #7882, #14276, #7800 ) ;
#6302=EDGE_LOOP ( 'NONE', ( #9915, #15519, #4500, #15637 ) ) ;
#6303=FACE_OUTER_BOUND ( 'NONE', #4621, .T. ) ;
#6306=CARTESIAN_POINT ( 'NONE',  ( 5.000000000000000000, 102.0000000000000142, 7.580410092413964129 ) ) ;
#6318=EDGE_CURVE ( 'NONE', #6916, #15230, #7967, .T. ) ;
#6320=ORIENTED_EDGE ( 'NONE', *, *, #9291, .F. ) ;
#6321=ORIENTED_EDGE ( 'NONE', *, *, #606, .F. ) ;
#6335=AXIS2_PLACEMENT_3D ( 'NONE', #12363, #15863, #4486 ) ;
#6352=DIRECTION ( 'NONE',  ( -6.938893903907231459E-18, 1.000000000000000000, 5.551115123125782702E-17 ) ) ;
#6396=ORIENTED_EDGE ( 'NONE', *, *, #213, .T. ) ;
#6417=ORIENTED_EDGE ( 'NONE', *, *, #8241, .T. ) ;
#6418=EDGE_CURVE ( 'NONE', #3981, #14778, #5641, .T. ) ;
#6420=ORIENTED_EDGE ( 'NONE', *, *, #8343, .F. ) ;
#6442=EDGE_CURVE ( 'NONE', #4234, #14778, #8753, .T. ) ;
#6461=CARTESIAN_POINT ( 'NONE',  ( 0.1743114854953164983, 100.0076106038165165, 5.000000000000000000 ) ) ;
#6463=VECTOR ( 'NONE', #8450, 1000.000000000000114 ) ;
#6467=FACE_OUTER_BOUND ( 'NONE', #10361, .T. ) ;
#6474=AXIS2_PLACEMENT_3D ( 'NONE', #14877, #7250, #660 ) ;
#6478=ORIENTED_EDGE ( 'NONE', *, *, #213, .F. ) ;
#6484=PLANE ( 'NONE',  #8609 ) ;
#6498=PLANE ( 'NONE',  #10161 ) ;
#6503=DIRECTION ( 'NONE',  ( -6.938893903907231459E-18, 1.000000000000000000, 5.551115123125782702E-17 ) ) ;
#6504=DIRECTION ( 'NONE',  ( -6.938893903907231459E-18, 1.000000000000000000, 5.551115123125782702E-17 ) ) ;
#6512=AXIS2_PLACEMENT_3D ( 'NONE', #4004, #6503, #2745 ) ;
#6536=VECTOR ( 'NONE', #7166, 1000.000000000000000 ) ;
#6543=STYLED_ITEM ( 'NONE', ( #4403 ), #8007 ) ;
#6545=CARTESIAN_POINT ( 'NONE',  ( -7.580410092413979228, 102.0000000000000142, -5.000000000000000000 ) ) ;
#6549=VECTOR ( 'NONE', #15980, 1000.000000000000000 ) ;
#6555=CARTESIAN_POINT ( 'NONE',  ( -5.000000000000000000, 92.00000000000001421, 0.000000000000000000 ) ) ;
#6556=CARTESIAN_POINT ( 'NONE',  ( 4.716203841691264387, 99.57974595388792238, -8.487905985326161584 ) ) ;
#6565=DIRECTION ( 'NONE',  ( -0.9993309688977879413, 0.03657341386592747462, 0.000000000000000000 ) ) ;
#6578=CONICAL_SURFACE ( 'NONE', #9227, 35.00000000000000711, 0.3490658503988666728 ) ;
#6600=ORIENTED_EDGE ( 'NONE', *, *, #11297, .F. ) ;
#6628=EDGE_CURVE ( 'NONE', #8437, #3904, #6930, .T. ) ;
#6636=CARTESIAN_POINT ( 'NONE',  ( -8.660254037844415720, 37.00000000000001421, -4.999999999999952038 ) ) ;
#6641=DIRECTION ( 'NONE',  ( 6.938893903907231459E-18, -1.000000000000000000, -5.551115123125782702E-17 ) ) ;
#6681=PRODUCT ( 'cutter assembly', 'cutter assembly', '', ( #14349 ) ) ;
#6684=CARTESIAN_POINT ( 'NONE',  ( 22.35235477796485171, 99.04060251627520017, -4.999999999999976019 ) ) ;
#6719=VECTOR ( 'NONE', #15781, 999.9999999999998863 ) ;
#6747=AXIS2_PLACEMENT_3D ( 'NONE', #11733, #335, #5434 ) ;
#6757=EDGE_LOOP ( 'NONE', ( #8083, #877, #8793, #10480, #6939 ) ) ;
#6766=CARTESIAN_POINT ( 'NONE',  ( -8.487905985326070990, 95.47132599478250370, -3.471325994782474389 ) ) ;
#6776=VECTOR ( 'NONE', #13854, 1000.000000000000000 ) ;
#6786=DIRECTION ( 'NONE',  ( -0.9777979793268661846, 0.2095497831645198317, 0.000000000000000000 ) ) ;
#6795=COLOUR_RGB ( '', 0.72549020, 0.75294118, 0.79215686) ;
#6802=CYLINDRICAL_SURFACE ( 'NONE', #10525, 45.00000000000000711 ) ;
#6803=VECTOR ( 'NONE', #8371, 1000.000000000000114 ) ;
#6838=ORIENTED_EDGE ( 'NONE', *, *, #14308, .T. ) ;
#6840=ORIENTED_EDGE ( 'NONE', *, *, #5021, .F. ) ;
#6841=ORIENTED_EDGE ( 'NONE', *, *, #2331, .T. ) ;
#6865=ORIENTED_EDGE ( 'NONE', *, *, #5330, .T. ) ;
#6894=ORIENTED_EDGE ( 'NONE', *, *, #7286, .F. ) ;
#6916=VERTEX_POINT ( 'NONE', #12643 ) ;
#6924=DIRECTION ( 'NONE',  ( 0.8660254037844362651, -8.780190904559507395E-17, -0.5000000000000042188 ) ) ;
#6930=LINE ( 'NONE', #4269, #3891 ) ;
#6937=EDGE_LOOP ( 'NONE', ( #5610, #14737 ) ) ;
#6939=ORIENTED_EDGE ( 'NONE', *, *, #7286, .T. ) ;
#6954=EDGE_LOOP ( 'NONE', ( #14572, #2478 ) ) ;
#6988=ORIENTED_EDGE ( 'NONE', *, *, #11109, .F. ) ;
#6989=EDGE_LOOP ( 'NONE', ( #13972, #467, #14488, #7179 ) ) ;
#6992=FACE_BOUND ( 'NONE', #6937, .T. ) ;
#6998=DIRECTION ( 'NONE',  ( -0.9361168066628589024, -0.08189960831908940642, -0.3420201433256691015 ) ) ;
#7018=VECTOR ( 'NONE', #1733, 1000.000000000000114 ) ;
#7030=AXIS2_PLACEMENT_3D ( 'NONE', #11309, #10063, #6158 ) ;
#7033=ORIENTED_EDGE ( 'NONE', *, *, #2049, .F. ) ;
#7034=EDGE_LOOP ( 'NONE', ( #7555, #13599, #9705, #15205 ) ) ;
#7045=EDGE_LOOP ( 'NONE', ( #6320, #6988, #6600, #14208 ) ) ;
#7049=AXIS2_PLACEMENT_3D ( 'NONE', #473, #1567, #9226 ) ;
#7050=ORIENTED_EDGE ( 'NONE', *, *, #15947, .T. ) ;
#7052=CARTESIAN_POINT ( 'NONE',  ( 1.034004556265705202E-14, 102.0000000000000142, 9.080892972013893782 ) ) ;
#7085=DIRECTION ( 'NONE',  ( -0.08715574274765824914, 0.9961946980917455452, 0.000000000000000000 ) ) ;
#7086=ADVANCED_FACE ( 'NONE', ( #14118 ), #11961, .F. ) ;
#7098=CARTESIAN_POINT ( 'NONE',  ( 7.580410092413998768, 99.32916037694960210, -5.000000000000000000 ) ) ;
#7106=CARTESIAN_POINT ( 'NONE',  ( -7.580410092413979228, 99.32916037694960210, -5.000000000000000000 ) ) ;
#7120=EDGE_LOOP ( 'NONE', ( #11308, #10341, #2475, #14945, #15875 ) ) ;
#7150=( BOUNDED_CURVE ( )  B_SPLINE_CURVE ( 3, ( #14957, #2486, #12796, #8727 ),
 .UNSPECIFIED., .F., .F. ) 
 B_SPLINE_CURVE_WITH_KNOTS ( ( 4, 4 ),
 ( 2.558501865821649623, 3.141592653589793116 ),
 .UNSPECIFIED. ) 
 CURVE ( )  GEOMETRIC_REPRESENTATION_ITEM ( )  RATIONAL_B_SPLINE_CURVE ( ( 1.000000000000000000, 0.9718672150731670900, 0.9718672150731670900, 1.000000000000000000 ) ) 
 REPRESENTATION_ITEM ( '' )  );
#7156=EDGE_LOOP ( 'NONE', ( #1225, #5904 ) ) ;
#7160=AXIS2_PLACEMENT_3D ( 'NONE', #2711, #5321, #12860 ) ;
#7166=DIRECTION ( 'NONE',  ( -6.938893903907231459E-18, 1.000000000000000000, 5.551115123125782702E-17 ) ) ;
#7176=EDGE_LOOP ( 'NONE', ( #5510, #3838, #1937, #3536, #7459 ) ) ;
#7178=EDGE_CURVE ( 'NONE', #2273, #15190, #2985, .T. ) ;
#7179=ORIENTED_EDGE ( 'NONE', *, *, #6318, .F. ) ;
#7202=EDGE_CURVE ( 'NONE', #7285, #2610, #12591, .T. ) ;
#7208=ORIENTED_EDGE ( 'NONE', *, *, #10278, .T. ) ;
#7223=CARTESIAN_POINT ( 'NONE',  ( -7.580410092413954359, 101.3368000520362813, 5.000000000000000000 ) ) ;
#7225=DIRECTION ( 'NONE',  ( -6.938893903907231459E-18, 1.000000000000000000, 5.551115123125782702E-17 ) ) ;
#7240=ADVANCED_FACE ( 'NONE', ( #13534, #2137 ), #14683, .T. ) ;
#7250=DIRECTION ( 'NONE',  ( -1.000000000000000000, 0.000000000000000000, 0.000000000000000000 ) ) ;
#7261=EDGE_LOOP ( 'NONE', ( #11367, #7208, #545, #4542 ) ) ;
#7282=EDGE_CURVE ( 'NONE', #58, #6916, #4492, .T. ) ;
#7285=VERTEX_POINT ( 'NONE', #12284 ) ;
#7286=EDGE_CURVE ( 'NONE', #894, #12156, #8222, .T. ) ;
#7301=VECTOR ( 'NONE', #13191, 1000.000000000000000 ) ;
#7312=DIRECTION ( 'NONE',  ( 6.938893903907231459E-18, -1.000000000000000000, -5.551115123125782702E-17 ) ) ;
#7349=PLANE ( 'NONE',  #14755 ) ;
#7361=CIRCLE ( 'NONE', #4176, 45.00000000000000711 ) ;
#7370=VECTOR ( 'NONE', #4005, 1000.000000000000114 ) ;
#7386=EDGE_CURVE ( 'NONE', #172, #16078, #16025, .T. ) ;
#7406=CARTESIAN_POINT ( 'NONE',  ( 9.657683769731223222, 91.78451504404918637, 2.612942168795361120 ) ) ;
#7411=DIRECTION ( 'NONE',  ( 0.000000000000000000, 0.000000000000000000, -1.000000000000000000 ) ) ;
#7449=DIRECTION ( 'NONE',  ( 6.938893903907231459E-18, -1.000000000000000000, -5.551115123125782702E-17 ) ) ;
#7459=ORIENTED_EDGE ( 'NONE', *, *, #6127, .T. ) ;
#7492=CARTESIAN_POINT ( 'NONE',  ( 0.000000000000000000, 102.0000000000000142, -5.000000000000000000 ) ) ;
#7511=VECTOR ( 'NONE', #2716, 1000.000000000000000 ) ;
#7529=( BOUNDED_CURVE ( )  B_SPLINE_CURVE ( 3, ( #948, #784, #6129, #16251 ),
 .UNSPECIFIED., .F., .F. ) 
 B_SPLINE_CURVE_WITH_KNOTS ( ( 4, 4 ),
 ( 5.700094519411438299, 6.866276094947727948 ),
 .UNSPECIFIED. ) 
 CURVE ( )  GEOMETRIC_REPRESENTATION_ITEM ( )  RATIONAL_B_SPLINE_CURVE ( ( 1.000000000000000000, 0.8898432210558864242, 0.8898432210558864242, 1.000000000000000000 ) ) 
 REPRESENTATION_ITEM ( '' )  );
#7537=ORIENTED_EDGE ( 'NONE', *, *, #10707, .F. ) ;
#7555=ORIENTED_EDGE ( 'NONE', *, *, #1717, .T. ) ;
#7600=ORIENTED_EDGE ( 'NONE', *, *, #15947, .F. ) ;
#7602=VECTOR ( 'NONE', #15665, 1000.000000000000000 ) ;
#7603=EDGE_LOOP ( 'NONE', ( #9359, #3230 ) ) ;
#7608=VECTOR ( 'NONE', #1750, 1000.000000000000000 ) ;
#7626=CYLINDRICAL_SURFACE ( 'NONE', #4958, 14.08089297201391155 ) ;
#7646=EDGE_CURVE ( 'NONE', #11207, #1716, #5244, .T. ) ;
#7692=DIRECTION ( 'NONE',  ( 0.000000000000000000, -1.541976423090494894E-16, -1.000000000000000000 ) ) ;
#7701=DIRECTION ( 'NONE',  ( -6.938893903907231459E-18, 1.000000000000000000, 5.551115123125782702E-17 ) ) ;
#7710=DIRECTION ( 'NONE',  ( -6.938893903907231459E-18, 1.000000000000000000, 5.551115123125782702E-17 ) ) ;
#7725=CARTESIAN_POINT ( 'NONE',  ( -5.000000000000000000, 96.75198296766782846, -7.580410092413988998 ) ) ;
#7745=EDGE_CURVE ( 'NONE', #9153, #9017, #8767, .T. ) ;
#7760=UNCERTAINTY_MEASURE_WITH_UNIT (LENGTH_MEASURE( 1.000000000000000082E-05 ), #3062, 'distance_accuracy_value', 'NONE');
#7788=FACE_OUTER_BOUND ( 'NONE', #7261, .T. ) ;
#7800=DIRECTION ( 'NONE',  ( -1.000000000000000000, 0.000000000000000000, -0.000000000000000000 ) ) ;
#7803=CARTESIAN_POINT ( 'NONE',  ( 9.262651381018932677E-15, 102.0000000000000142, -9.080892972013931086 ) ) ;
#7820=SURFACE_STYLE_FILL_AREA ( #10081 ) ;
#7842=AXIS2_PLACEMENT_3D ( 'NONE', #965, #13602, #2053 ) ;
#7854=VECTOR ( 'NONE', #1460, 999.9999999999998863 ) ;
#7859=LINE ( 'NONE', #6461, #10209 ) ;
#7874=AXIS2_PLACEMENT_3D ( 'NONE', #8488, #1758, #3676 ) ;
#7882=CARTESIAN_POINT ( 'NONE',  ( 0.000000000000000000, 0.000000000000000000, -5.000000000000000000 ) ) ;
#7883=ORIENTED_EDGE ( 'NONE', *, *, #6418, .T. ) ;
#7918=CARTESIAN_POINT ( 'NONE',  ( -5.000000000000000000, 99.58041009241402719, -7.580410092413988998 ) ) ;
#7967=( BOUNDED_CURVE ( )  B_SPLINE_CURVE ( 3, ( #13739, #14724, #9927, #16237 ),
 .UNSPECIFIED., .F., .F. ) 
 B_SPLINE_CURVE_WITH_KNOTS ( ( 4, 4 ),
 ( 5.700094519411438299, 6.866276094947727948 ),
 .UNSPECIFIED. ) 
 CURVE ( )  GEOMETRIC_REPRESENTATION_ITEM ( )  RATIONAL_B_SPLINE_CURVE ( ( 1.000000000000000000, 0.8898432210558864242, 0.8898432210558864242, 1.000000000000000000 ) ) 
 REPRESENTATION_ITEM ( '' )  );
#7975=DIRECTION ( 'NONE',  ( -6.938893903907231459E-18, 1.000000000000000000, 5.551115123125782702E-17 ) ) ;
#7992=LINE ( 'NONE', #11899, #4688 ) ;
#7995=CARTESIAN_POINT ( 'NONE',  ( 0.000000000000000000, 102.0000000000000142, 5.000000000000000000 ) ) ;
#8007=ADVANCED_BREP_SHAPE_REPRESENTATION ( '', ( #8709, #15812 ), #3617 ) ;
#8045=CARTESIAN_POINT ( 'NONE',  ( -5.000000000000000000, 92.00000000000001421, 0.000000000000000000 ) ) ;
#8054=CARTESIAN_POINT ( 'NONE',  ( 9.574901606694759531E-15, 52.00000000000001421, 34.99999999999999289 ) ) ;
#8058=FACE_OUTER_BOUND ( 'NONE', #4779, .T. ) ;
#8062=VERTEX_POINT ( 'NONE', #13083 ) ;
#8073=DIRECTION ( 'NONE',  ( 0.08715574274765797158, 0.9961946980917455452, -0.000000000000000000 ) ) ;
#8079=VECTOR ( 'NONE', #7701, 1000.000000000000000 ) ;
#8083=ORIENTED_EDGE ( 'NONE', *, *, #1120, .T. ) ;
#8085=EDGE_CURVE ( 'NONE', #15764, #12729, #8090, .T. ) ;
#8090=LINE ( 'NONE', #1688, #14180 ) ;
#8104=ORIENTED_EDGE ( 'NONE', *, *, #12874, .F. ) ;
#8123=EDGE_CURVE ( 'NONE', #172, #5355, #5964, .T. ) ;
#8130=LINE ( 'NONE', #8045, #1786 ) ;
#8143=ADVANCED_FACE ( 'NONE', ( #4762 ), #2402, .F. ) ;
#8177=ORIENTED_EDGE ( 'NONE', *, *, #10399, .T. ) ;
#8211=ADVANCED_FACE ( 'NONE', ( #12475 ), #15038, .T. ) ;
#8222=LINE ( 'NONE', #13288, #14422 ) ;
#8230=EDGE_LOOP ( 'NONE', ( #8251, #15609, #5953, #3538 ) ) ;
#8241=EDGE_CURVE ( 'NONE', #9035, #9419, #15420, .T. ) ;
#8245=FACE_OUTER_BOUND ( 'NONE', #622, .T. ) ;
#8251=ORIENTED_EDGE ( 'NONE', *, *, #2008, .F. ) ;
#8276=LINE ( 'NONE', #11936, #16083 ) ;
#8318=PLANE ( 'NONE',  #2364 ) ;
#8330=CARTESIAN_POINT ( 'NONE',  ( -1.688807283342573573, 101.8522485078275253, 9.657683769731223222 ) ) ;
#8332=LINE ( 'NONE', #13396, #11582 ) ;
#8336=EDGE_CURVE ( 'NONE', #8062, #10751, #12605, .T. ) ;
#8343=EDGE_CURVE ( 'NONE', #16281, #332, #7859, .T. ) ;
#8349=EDGE_CURVE ( 'NONE', #12433, #16149, #4679, .T. ) ;
#8363=ORIENTED_EDGE ( 'NONE', *, *, #7178, .F. ) ;
#8364=EDGE_CURVE ( 'NONE', #14778, #10814, #12530, .T. ) ;
#8371=DIRECTION ( 'NONE',  ( 0.000000000000000000, -0.7890408728378107694, -0.6143407043256581268 ) ) ;
#8415=PRODUCT_DEFINITION_CONTEXT ( 'detailed design', #10053, 'design' ) ;
#8437=VERTEX_POINT ( 'NONE', #14408 ) ;
#8450=DIRECTION ( 'NONE',  ( 0.3420201433256697121, 0.6644630243886755494, -0.6644630243886733290 ) ) ;
#8459=DIRECTION ( 'NONE',  ( 6.938893903907231459E-18, -1.000000000000000000, -5.551115123125782702E-17 ) ) ;
#8466=CARTESIAN_POINT ( 'NONE',  ( -7.580410092413979228, 101.3368000520362813, -5.000000000000000000 ) ) ;
#8485=FACE_OUTER_BOUND ( 'NONE', #3295, .T. ) ;
#8488=CARTESIAN_POINT ( 'NONE',  ( 9.657683769731171708, 93.19872860642226442, 1.198728606422249987 ) ) ;
#8497=ORIENTED_EDGE ( 'NONE', *, *, #4317, .T. ) ;
#8502=CARTESIAN_POINT ( 'NONE',  ( 5.000000000000000000, 107.2206331336081462, 16.63484669598117094 ) ) ;
#8529=EDGE_CURVE ( 'NONE', #2458, #3153, #14970, .T. ) ;
#8539=EDGE_CURVE ( 'NONE', #15190, #1407, #4658, .T. ) ;
#8560=DIRECTION ( 'NONE',  ( 1.000000000000000000, 0.000000000000000000, 0.000000000000000000 ) ) ;
#8570=ORIENTED_EDGE ( 'NONE', *, *, #8364, .T. ) ;
#8609=AXIS2_PLACEMENT_3D ( 'NONE', #143, #1232, #1143 ) ;
#8610=ADVANCED_FACE ( 'NONE', ( #3596 ), #3260, .F. ) ;
#8616=DIRECTION ( 'NONE',  ( 0.000000000000000000, -5.551115123125782702E-17, 1.000000000000000000 ) ) ;
#8627=EDGE_CURVE ( 'NONE', #2051, #10856, #10237, .T. ) ;
#8630=ORIENTED_EDGE ( 'NONE', *, *, #15556, .F. ) ;
#8637=EDGE_CURVE ( 'NONE', #10236, #2273, #13928, .T. ) ;
#8638=DIRECTION ( 'NONE',  ( -0.9361168066628590134, 0.08189960831908912886, -0.3420201433256691570 ) ) ;
#8654=ORIENTED_EDGE ( 'NONE', *, *, #14649, .T. ) ;
#8655=VECTOR ( 'NONE', #8852, 1000.000000000000000 ) ;
#8658=CARTESIAN_POINT ( 'NONE',  ( 9.574901606694759531E-15, 52.00000000000001421, -2.191293403013901163E-14 ) ) ;
#8689=DIRECTION ( 'NONE',  ( -0.08715574274765824914, 0.9961946980917455452, 0.000000000000000000 ) ) ;
#8709=MANIFOLD_SOLID_BREP ( 'Boss-Extrude5', #4967 ) ;
#8715=CARTESIAN_POINT ( 'NONE',  ( 9.657683769731161050, 93.19872860642226442, 1.198728606422247323 ) ) ;
#8727=CARTESIAN_POINT ( 'NONE',  ( 9.253960653386475815E-15, 98.25246584726779986, -9.080892972013931086 ) ) ;
#8728=CARTESIAN_POINT ( 'NONE',  ( 9.397478011314830142E-15, 45.00000000000000711, -45.00000000000002842 ) ) ;
#8753=LINE ( 'NONE', #1422, #9485 ) ;
#8767=LINE ( 'NONE', #5211, #11279 ) ;
#8793=ORIENTED_EDGE ( 'NONE', *, *, #1717, .F. ) ;
#8800=ORIENTED_EDGE ( 'NONE', *, *, #13511, .T. ) ;
#8804=FACE_OUTER_BOUND ( 'NONE', #7176, .T. ) ;
#8807=LINE ( 'NONE', #1071, #14681 ) ;
#8839=ADVANCED_FACE ( 'NONE', ( #9643 ), #4579, .F. ) ;
#8852=DIRECTION ( 'NONE',  ( -0.000000000000000000, -0.7890408728378112135, 0.6143407043256575717 ) ) ;
#8864=CARTESIAN_POINT ( 'NONE',  ( 1.036604930454412972E-14, 98.25246584726775723, 9.080892972013893782 ) ) ;
#8885=AXIS2_PLACEMENT_3D ( 'NONE', #7406, #3666, #14785 ) ;
#8923=AXIS2_PLACEMENT_3D ( 'NONE', #15504, #14173, #1008 ) ;
#8926=ORIENTED_EDGE ( 'NONE', *, *, #4317, .F. ) ;
#8935=AXIS2_PLACEMENT_3D ( 'NONE', #3528, #3273, #10925 ) ;
#8940=VECTOR ( 'NONE', #10313, 1000.000000000000114 ) ;
#8951=CARTESIAN_POINT ( 'NONE',  ( 1.034642314881058238E-14, 101.0808929720139417, 9.080892972013893782 ) ) ;
#8966=CARTESIAN_POINT ( 'NONE',  ( 4.883629682448357379, 95.00500682027384869, 5.000000000000000888 ) ) ;
#8976=LINE ( 'NONE', #12964, #9831 ) ;
#8990=ADVANCED_FACE ( 'NONE', ( #10223 ), #6484, .F. ) ;
#8997=ORIENTED_EDGE ( 'NONE', *, *, #5569, .F. ) ;
#9017=VERTEX_POINT ( 'NONE', #16372 ) ;
#9035=VERTEX_POINT ( 'NONE', #2400 ) ;
#9067=DIRECTION ( 'NONE',  ( 0.000000000000000000, 8.780190904559502465E-17, 1.000000000000000000 ) ) ;
#9069=CARTESIAN_POINT ( 'NONE',  ( 1.036604930454412972E-14, 98.25246584726775723, 9.080892972013893782 ) ) ;
#9076=CARTESIAN_POINT ( 'NONE',  ( 9.297345850538470396E-15, 92.00000000000001421, -1.969248798088869855E-14 ) ) ;
#9100=LINE ( 'NONE', #5059, #12372 ) ;
#9113=ORIENTED_EDGE ( 'NONE', *, *, #815, .T. ) ;
#9115=PLANE ( 'NONE',  #8923 ) ;
#9130=ORIENTED_EDGE ( 'NONE', *, *, #1049, .T. ) ;
#9131=ORIENTED_EDGE ( 'NONE', *, *, #4713, .F. ) ;
#9136=AXIS2_PLACEMENT_3D ( 'NONE', #558, #15372, #9067 ) ;
#9151=AXIS2_PLACEMENT_3D ( 'NONE', #14953, #16376, #5914 ) ;
#9153=VERTEX_POINT ( 'NONE', #1644 ) ;
#9174=VECTOR ( 'NONE', #16348, 999.9999999999998863 ) ;
#9187=LINE ( 'NONE', #5547, #15558 ) ;
#9200=AXIS2_PLACEMENT_3D ( 'NONE', #15140, #6352, #11418 ) ;
#9226=DIRECTION ( 'NONE',  ( 0.000000000000000000, -0.7071067811865487940, 0.7071067811865463515 ) ) ;
#9227=AXIS2_PLACEMENT_3D ( 'NONE', #16016, #8459, #14761 ) ;
#9287=FACE_OUTER_BOUND ( 'NONE', #16029, .T. ) ;
#9291=EDGE_CURVE ( 'NONE', #9644, #1716, #9464, .T. ) ;
#9312=FACE_OUTER_BOUND ( 'NONE', #9482, .T. ) ;
#9337=CARTESIAN_POINT ( 'NONE',  ( -5.000000000000000000, 107.2206331336081320, -16.63484669598115673 ) ) ;
#9356=ADVANCED_FACE ( 'NONE', ( #2976 ), #12963, .T. ) ;
#9359=ORIENTED_EDGE ( 'NONE', *, *, #10707, .T. ) ;
#9380=ADVANCED_FACE ( 'NONE', ( #3394 ), #11039, .T. ) ;
#9419=VERTEX_POINT ( 'NONE', #12277 ) ;
#9464=LINE ( 'NONE', #231, #15537 ) ;
#9466=DIRECTION ( 'NONE',  ( 0.3420201433256698231, 0.6644630243886754384, -0.6644630243886734400 ) ) ;
#9475=( NAMED_UNIT ( * ) SI_UNIT ( $, .STERADIAN. ) SOLID_ANGLE_UNIT ( ) );
#9482=EDGE_LOOP ( 'NONE', ( #5334, #15303 ) ) ;
#9485=VECTOR ( 'NONE', #16407, 1000.000000000000000 ) ;
#9486=ORIENTED_EDGE ( 'NONE', *, *, #1120, .F. ) ;
#9514=EDGE_CURVE ( 'NONE', #10158, #2051, #12115, .T. ) ;
#9537=CARTESIAN_POINT ( 'NONE',  ( -1.790468199911974034, 98.25246584726781407, -9.080892972013931086 ) ) ;
#9550=CARTESIAN_POINT ( 'NONE',  ( -8.487905985326078095, 95.47132599478250370, -3.471325994782476609 ) ) ;
#9570=CARTESIAN_POINT ( 'NONE',  ( 9.574901606694759531E-15, 52.00000000000001421, -2.191293403013901163E-14 ) ) ;
#9622=FACE_OUTER_BOUND ( 'NONE', #2999, .T. ) ;
#9637=EDGE_CURVE ( 'NONE', #10236, #1407, #11287, .T. ) ;
#9643=FACE_OUTER_BOUND ( 'NONE', #7120, .T. ) ;
#9644=VERTEX_POINT ( 'NONE', #1375 ) ;
#9648=LINE ( 'NONE', #13626, #6536 ) ;
#9660=CARTESIAN_POINT ( 'NONE',  ( 9.574901606694759531E-15, 52.00000000000001421, 34.99999999999999289 ) ) ;
#9701=ORIENTED_EDGE ( 'NONE', *, *, #6628, .F. ) ;
#9705=ORIENTED_EDGE ( 'NONE', *, *, #13316, .F. ) ;
#9706=AXIS2_PLACEMENT_3D ( 'NONE', #12346, #8689, #13427 ) ;
#9710=LINE ( 'NONE', #7052, #13722 ) ;
#9754=AXIS2_PLACEMENT_3D ( 'NONE', #9076, #6504, #1163 ) ;
#9758=VERTEX_POINT ( 'NONE', #15011 ) ;
#9769=DIRECTION ( 'NONE',  ( 0.3213938048432687378, 0.5817472440052507965, 0.7471788047720987480 ) ) ;
#9800=PLANE ( 'NONE',  #11368 ) ;
#9815=VECTOR ( 'NONE', #2058, 1000.000000000000114 ) ;
#9827=FACE_OUTER_BOUND ( 'NONE', #1026, .T. ) ;
#9831=VECTOR ( 'NONE', #15276, 1000.000000000000000 ) ;
#9836=ORIENTED_EDGE ( 'NONE', *, *, #8085, .F. ) ;
#9839=CARTESIAN_POINT ( 'NONE',  ( -1.688807283342575793, 101.8522485078275253, 9.657683769731228551 ) ) ;
#9888=ADVANCED_FACE ( 'NONE', ( #11935 ), #6802, .T. ) ;
#9915=ORIENTED_EDGE ( 'NONE', *, *, #15238, .T. ) ;
#9927=CARTESIAN_POINT ( 'NONE',  ( 9.642970592016647302, 99.14870971539799882, -1.872989114519519882 ) ) ;
#9936=EDGE_CURVE ( 'NONE', #14188, #3704, #10539, .T. ) ;
#9954=CARTESIAN_POINT ( 'NONE',  ( 1.490838860747792127E-14, 45.00000000000002132, 44.99999999999998579 ) ) ;
#9956=AXIS2_PLACEMENT_3D ( 'NONE', #1065, #13378, #899 ) ;
#9968=ADVANCED_FACE ( 'NONE', ( #9287, #11615 ), #10366, .F. ) ;
#9974=ADVANCED_FACE ( 'NONE', ( #15425, #4045 ), #9115, .T. ) ;
#9993=CARTESIAN_POINT ( 'NONE',  ( -7.580410092413954359, 99.32916037694960210, 5.000000000000000000 ) ) ;
#10050=VECTOR ( 'NONE', #16439, 1000.000000000000000 ) ;
#10053=APPLICATION_CONTEXT ( 'automotive_design' ) ;
#10063=DIRECTION ( 'NONE',  ( 0.000000000000000000, 0.7071067811865463515, -0.7071067811865487940 ) ) ;
#10064=CARTESIAN_POINT ( 'NONE',  ( 5.000000000000000000, 0.000000000000000000, 0.000000000000000000 ) ) ;
#10066=DIRECTION ( 'NONE',  ( 0.000000000000000000, 1.541976423090494894E-16, 1.000000000000000000 ) ) ;
#10068=CARTESIAN_POINT ( 'NONE',  ( 1.875620865444973696E-15, 37.00000000000001421, -3.248670634687016947E-15 ) ) ;
#10070=CARTESIAN_POINT ( 'NONE',  ( 1.105645237078933619E-14, 92.00000000000001421, 14.08089297201389378 ) ) ;
#10081=FILL_AREA_STYLE ('',( #14129 ) ) ;
#10110=CARTESIAN_POINT ( 'NONE',  ( -5.000000000000000000, 32.40304740096967606, 41.61750739262920717 ) ) ;
#10113=SHAPE_REPRESENTATION ( 'cutter assembly', ( #15812 ), #3617 ) ;
#10138=EDGE_LOOP ( 'NONE', ( #11538, #11968 ) ) ;
#10158=VERTEX_POINT ( 'NONE', #8502 ) ;
#10161=AXIS2_PLACEMENT_3D ( 'NONE', #15376, #3999, #2738 ) ;
#10209=VECTOR ( 'NONE', #15171, 1000.000000000000000 ) ;
#10219=ORIENTED_EDGE ( 'NONE', *, *, #5489, .F. ) ;
#10222=EDGE_CURVE ( 'NONE', #12433, #3981, #5279, .T. ) ;
#10223=FACE_OUTER_BOUND ( 'NONE', #4086, .T. ) ;
#10228=CARTESIAN_POINT ( 'NONE',  ( 5.000000000000000000, 96.75198296766781425, 7.580410092413965017 ) ) ;
#10236=VERTEX_POINT ( 'NONE', #2593 ) ;
#10237=LINE ( 'NONE', #12808, #2519 ) ;
#10278=EDGE_CURVE ( 'NONE', #9153, #15764, #13887, .T. ) ;
#10291=PLANE ( 'NONE',  #10523 ) ;
#10313=DIRECTION ( 'NONE',  ( 0.9993309688977879413, -0.03657341386592747462, 0.000000000000000000 ) ) ;
#10322=ORIENTED_EDGE ( 'NONE', *, *, #11803, .T. ) ;
#10341=ORIENTED_EDGE ( 'NONE', *, *, #14628, .T. ) ;
#10350=DIRECTION ( 'NONE',  ( -5.069245582283711292E-17, -1.000000000000000000, 8.780190904559502465E-17 ) ) ;
#10361=EDGE_LOOP ( 'NONE', ( #6840, #12216, #12468, #3281 ) ) ;
#10365=LINE ( 'NONE', #10917, #15567 ) ;
#10366=PLANE ( 'NONE',  #4406 ) ;
#10367=CARTESIAN_POINT ( 'NONE',  ( 9.297345850538470396E-15, 92.00000000000001421, -1.969248798088869855E-14 ) ) ;
#10373=FACE_OUTER_BOUND ( 'NONE', #6757, .T. ) ;
#10387=EDGE_CURVE ( 'NONE', #58, #12729, #7992, .T. ) ;
#10399=EDGE_CURVE ( 'NONE', #16281, #11207, #5668, .T. ) ;
#10403=( BOUNDED_CURVE ( )  B_SPLINE_CURVE ( 3, ( #12947, #11693, #4047, #10623 ),
 .UNSPECIFIED., .F., .T. ) 
 B_SPLINE_CURVE_WITH_KNOTS ( ( 4, 4 ),
 ( 2.558501865821650068, 3.141592653589793116 ),
 .UNSPECIFIED. ) 
 CURVE ( )  GEOMETRIC_REPRESENTATION_ITEM ( )  RATIONAL_B_SPLINE_CURVE ( ( 1.000000000000000000, 0.9718672150731670900, 0.9718672150731670900, 1.000000000000000000 ) ) 
 REPRESENTATION_ITEM ( '' )  );
#10446=ORIENTED_EDGE ( 'NONE', *, *, #12513, .F. ) ;
#10447=CARTESIAN_POINT ( 'NONE',  ( -7.580410092413954359, 99.32916037694960210, 5.000000000000000000 ) ) ;
#10472=LINE ( 'NONE', #1813, #757 ) ;
#10480=ORIENTED_EDGE ( 'NONE', *, *, #4528, .F. ) ;
#10488=PLANE ( 'NONE',  #2290 ) ;
#10491=EDGE_CURVE ( 'NONE', #332, #12784, #9648, .T. ) ;
#10499=DIRECTION ( 'NONE',  ( -6.938893903907231459E-18, 1.000000000000000000, 5.551115123125782702E-17 ) ) ;
#10504=CARTESIAN_POINT ( 'NONE',  ( -3.505380114644267575, 100.5662537783984334, -8.566253778398381868 ) ) ;
#10523=AXIS2_PLACEMENT_3D ( 'NONE', #15097, #12608, #3724 ) ;
#10525=AXIS2_PLACEMENT_3D ( 'NONE', #457, #4220, #536 ) ;
#10537=EDGE_LOOP ( 'NONE', ( #11030, #7537, #8497, #10322 ) ) ;
#10539=LINE ( 'NONE', #6555, #7854 ) ;
#10573=ORIENTED_EDGE ( 'NONE', *, *, #6123, .F. ) ;
#10582=CARTESIAN_POINT ( 'NONE',  ( -0.1743114854953159432, 100.0076106038165165, 5.000000000000000000 ) ) ;
#10609=LINE ( 'NONE', #15822, #16351 ) ;
#10616=VERTEX_POINT ( 'NONE', #12303 ) ;
#10623=CARTESIAN_POINT ( 'NONE',  ( 9.234334497652928468E-15, 101.0808929720139702, -9.080892972013931086 ) ) ;
#10634=ORIENTED_EDGE ( 'NONE', *, *, #11535, .F. ) ;
#10648=CARTESIAN_POINT ( 'NONE',  ( -49.72257916183962578, 96.64601816452537264, -5.000000000000000000 ) ) ;
#10660=DIRECTION ( 'NONE',  ( 0.3420201433256698231, 0.6644630243886754384, -0.6644630243886734400 ) ) ;
#10672=EDGE_LOOP ( 'NONE', ( #10219, #9130, #548, #11653, #11869 ) ) ;
#10694=EDGE_CURVE ( 'NONE', #9644, #16281, #3502, .T. ) ;
#10707=EDGE_CURVE ( 'NONE', #13593, #5951, #12375, .T. ) ;
#10717=SURFACE_STYLE_FILL_AREA ( #2825 ) ;
#10735=CARTESIAN_POINT ( 'NONE',  ( -48.69930661242911185, 95.73172307475269349, -7.581784256837400982 ) ) ;
#10739=EDGE_CURVE ( 'NONE', #8437, #9035, #3990, .T. ) ;
#10751=VERTEX_POINT ( 'NONE', #12720 ) ;
#10782=SHAPE_DEFINITION_REPRESENTATION ( #3082, #10113 ) ;
#10787=AXIS2_PLACEMENT_3D ( 'NONE', #16239, #9769, #13574 ) ;
#10814=VERTEX_POINT ( 'NONE', #11312 ) ;
#10847=FACE_OUTER_BOUND ( 'NONE', #13258, .T. ) ;
#10851=ORIENTED_EDGE ( 'NONE', *, *, #11616, .T. ) ;
#10856=VERTEX_POINT ( 'NONE', #10228 ) ;
#10889=EDGE_LOOP ( 'NONE', ( #6420, #8177, #16415, #2560 ) ) ;
#10901=DIRECTION ( 'NONE',  ( 6.938893903907231459E-18, -1.000000000000000000, -5.551115123125782702E-17 ) ) ;
#10912=UNCERTAINTY_MEASURE_WITH_UNIT (LENGTH_MEASURE( 1.000000000000000082E-05 ), #1575, 'distance_accuracy_value', 'NONE');
#10917=CARTESIAN_POINT ( 'NONE',  ( -5.000000000000000000, 102.0000000000000142, -7.580410092413988998 ) ) ;
#10925=DIRECTION ( 'NONE',  ( 0.9361168066628590134, -0.08189960831908912886, 0.3420201433256691570 ) ) ;
#11013=VECTOR ( 'NONE', #15499, 1000.000000000000000 ) ;
#11030=ORIENTED_EDGE ( 'NONE', *, *, #12809, .F. ) ;
#11039=CYLINDRICAL_SURFACE ( 'NONE', #7842, 14.08089297201391155 ) ;
#11044=CARTESIAN_POINT ( 'NONE',  ( 0.000000000000000000, 102.0000000000000142, 5.000000000000000000 ) ) ;
#11045=CARTESIAN_POINT ( 'NONE',  ( -9.642970592016627762, 101.1563493904846780, -1.872989114519522547 ) ) ;
#11047=VECTOR ( 'NONE', #2190, 1000.000000000000000 ) ;
#11063=AXIS2_PLACEMENT_3D ( 'NONE', #13869, #12635, #10066 ) ;
#11073=DIRECTION ( 'NONE',  ( 0.000000000000000000, 0.000000000000000000, 1.000000000000000000 ) ) ;
#11076=DIRECTION ( 'NONE',  ( 0.08715574274765797158, 0.9961946980917455452, -0.000000000000000000 ) ) ;
#11108=EDGE_LOOP ( 'NONE', ( #6478, #5448, #5163, #624 ) ) ;
#11109=EDGE_CURVE ( 'NONE', #16226, #9644, #8332, .T. ) ;
#11124=VERTEX_POINT ( 'NONE', #437 ) ;
#11164=FACE_OUTER_BOUND ( 'NONE', #7034, .T. ) ;
#11195=EDGE_LOOP ( 'NONE', ( #14863, #6036, #4330, #6396, #13578 ) ) ;
#11199=EDGE_CURVE ( 'NONE', #2051, #3882, #4201, .T. ) ;
#11207=VERTEX_POINT ( 'NONE', #11828 ) ;
#11224=ORIENTED_EDGE ( 'NONE', *, *, #2331, .F. ) ;
#11235=CARTESIAN_POINT ( 'NONE',  ( 9.253960653386475815E-15, 98.25246584726779986, -9.080892972013931086 ) ) ;
#11236=DIRECTION ( 'NONE',  ( 5.069245582283711292E-17, 1.000000000000000000, -8.780190904559502465E-17 ) ) ;
#11250=LINE ( 'NONE', #9839, #431 ) ;
#11279=VECTOR ( 'NONE', #3710, 1000.000000000000000 ) ;
#11283=ORIENTED_EDGE ( 'NONE', *, *, #606, .T. ) ;
#11287=LINE ( 'NONE', #12775, #9174 ) ;
#11297=EDGE_CURVE ( 'NONE', #982, #16226, #11250, .T. ) ;
#11304=ADVANCED_FACE ( 'NONE', ( #6019 ), #7349, .T. ) ;
#11308=ORIENTED_EDGE ( 'NONE', *, *, #13316, .T. ) ;
#11309=CARTESIAN_POINT ( 'NONE',  ( 5.000000000000000000, 90.58578643762692195, 1.414213562373097588 ) ) ;
#11312=CARTESIAN_POINT ( 'NONE',  ( 5.000000000000000000, 99.58041009241399877, 7.580410092413963241 ) ) ;
#11316=LINE ( 'NONE', #15044, #1204 ) ;
#11367=ORIENTED_EDGE ( 'NONE', *, *, #7745, .F. ) ;
#11368=AXIS2_PLACEMENT_3D ( 'NONE', #9550, #13604, #9466 ) ;
#11388=ORIENTED_EDGE ( 'NONE', *, *, #11199, .T. ) ;
#11392=PLANE ( 'NONE',  #3984 ) ;
#11393=CIRCLE ( 'NONE', #4228, 24.08089297201390977 ) ;
#11397=DIRECTION ( 'NONE',  ( 0.000000000000000000, 0.000000000000000000, 1.000000000000000000 ) ) ;
#11418=DIRECTION ( 'NONE',  ( 0.000000000000000000, 0.000000000000000000, 1.000000000000000000 ) ) ;
#11428=ORIENTED_EDGE ( 'NONE', *, *, #6418, .F. ) ;
#11455=CARTESIAN_POINT ( 'NONE',  ( 5.000000000000000000, 126.6482322781408953, -36.06244584051386681 ) ) ;
#11461=EDGE_LOOP ( 'NONE', ( #5100, #9701, #962, #6417 ) ) ;
#11492=CARTESIAN_POINT ( 'NONE',  ( -5.000000000000000000, 99.58041009241398456, 7.580410092413952583 ) ) ;
#11519=VECTOR ( 'NONE', #7312, 1000.000000000000000 ) ;
#11535=EDGE_CURVE ( 'NONE', #2312, #10158, #11651, .T. ) ;
#11538=ORIENTED_EDGE ( 'NONE', *, *, #11616, .F. ) ;
#11543=DIRECTION ( 'NONE',  ( -1.000000000000000000, 0.000000000000000000, 0.000000000000000000 ) ) ;
#11566=CARTESIAN_POINT ( 'NONE',  ( -5.000000000000000000, 102.0000000000000142, 7.580410092413950807 ) ) ;
#11582=VECTOR ( 'NONE', #15813, 1000.000000000000227 ) ;
#11615=FACE_BOUND ( 'NONE', #16126, .T. ) ;
#11616=EDGE_CURVE ( 'NONE', #2610, #7285, #15314, .T. ) ;
#11629=VECTOR ( 'NONE', #15681, 1000.000000000000000 ) ;
#11636=DIRECTION ( 'NONE',  ( -0.9361168066628589024, -0.08189960831908939254, -0.3420201433256691570 ) ) ;
#11641=CARTESIAN_POINT ( 'NONE',  ( 9.366734789577542680E-15, 82.00000000000001421, -2.024759949320127682E-14 ) ) ;
#11651=LINE ( 'NONE', #12658, #7370 ) ;
#11653=ORIENTED_EDGE ( 'NONE', *, *, #12330, .T. ) ;
#11693=CARTESIAN_POINT ( 'NONE',  ( 3.505380114644272460, 100.5662537783984192, -8.566253778398381868 ) ) ;
#11717=( NAMED_UNIT ( * ) PLANE_ANGLE_UNIT ( ) SI_UNIT ( $, .RADIAN. ) );
#11733=CARTESIAN_POINT ( 'NONE',  ( 1.875620865444973696E-15, 37.00000000000001421, -3.248670634687016947E-15 ) ) ;
#11737=DIRECTION ( 'NONE',  ( 5.069245582283711292E-17, 1.000000000000000000, -8.780190904559503697E-17 ) ) ;
#11743=ORIENTED_EDGE ( 'NONE', *, *, #11109, .T. ) ;
#11766=ORIENTED_EDGE ( 'NONE', *, *, #9514, .T. ) ;
#11782=CARTESIAN_POINT ( 'NONE',  ( 9.332040320058006538E-15, 92.00000000000001421, -14.08089297201393109 ) ) ;
#11803=EDGE_CURVE ( 'NONE', #2563, #12657, #7361, .T. ) ;
#11822=ADVANCED_FACE ( 'NONE', ( #6992, #1745 ), #10488, .T. ) ;
#11828=CARTESIAN_POINT ( 'NONE',  ( -41.63290517038959848, 96.34995309285439191, -5.000000000000000000 ) ) ;
#11868=ORIENTED_EDGE ( 'NONE', *, *, #4641, .T. ) ;
#11869=ORIENTED_EDGE ( 'NONE', *, *, #10222, .F. ) ;
#11899=CARTESIAN_POINT ( 'NONE',  ( 0.000000000000000000, 102.0000000000000142, 5.000000000000000000 ) ) ;
#11902=( BOUNDED_CURVE ( )  B_SPLINE_CURVE ( 3, ( #7106, #14413, #12162, #10447 ),
 .UNSPECIFIED., .F., .F. ) 
 B_SPLINE_CURVE_WITH_KNOTS ( ( 4, 4 ),
 ( 5.700094519411444516, 6.866276094947734165 ),
 .UNSPECIFIED. ) 
 CURVE ( )  GEOMETRIC_REPRESENTATION_ITEM ( )  RATIONAL_B_SPLINE_CURVE ( ( 1.000000000000000000, 0.8898432210558864242, 0.8898432210558864242, 1.000000000000000000 ) ) 
 REPRESENTATION_ITEM ( '' )  );
#11903=ADVANCED_FACE ( 'NONE', ( #4759 ), #16208, .T. ) ;
#11932=VERTEX_POINT ( 'NONE', #2071 ) ;
#11935=FACE_OUTER_BOUND ( 'NONE', #4737, .T. ) ;
#11936=CARTESIAN_POINT ( 'NONE',  ( -5.000000000000000000, 61.36844557917451937, -47.78096468550220521 ) ) ;
#11945=ADVANCED_FACE ( 'NONE', ( #5994 ), #14506, .T. ) ;
#11960=( NAMED_UNIT ( * ) SI_UNIT ( $, .STERADIAN. ) SOLID_ANGLE_UNIT ( ) );
#11961=PLANE ( 'NONE',  #9136 ) ;
#11968=ORIENTED_EDGE ( 'NONE', *, *, #7202, .F. ) ;
#11974=ORIENTED_EDGE ( 'NONE', *, *, #1309, .T. ) ;
#11977=DIRECTION ( 'NONE',  ( 0.9961946980917455452, -0.08715574274765795770, 0.000000000000000000 ) ) ;
#12008=EDGE_LOOP ( 'NONE', ( #4690, #11388, #5574, #3166, #11974 ) ) ;
#12029=CARTESIAN_POINT ( 'NONE',  ( -5.000000000000000000, 102.2474899284556500, -10.24748992845560380 ) ) ;
#12049=CARTESIAN_POINT ( 'NONE',  ( 9.574901606694759531E-15, 52.00000000000001421, -2.191293403013901479E-14 ) ) ;
#12065=DIRECTION ( 'NONE',  ( -0.5000000000000042188, -0.000000000000000000, -0.8660254037844362651 ) ) ;
#12110=VERTEX_POINT ( 'NONE', #7803 ) ;
#12115=LINE ( 'NONE', #4560, #6803 ) ;
#12156=VERTEX_POINT ( 'NONE', #14110 ) ;
#12157=CARTESIAN_POINT ( 'NONE',  ( 5.000000000000000000, 92.00000000000001421, 0.000000000000000000 ) ) ;
#12162=CARTESIAN_POINT ( 'NONE',  ( -9.642970592016617104, 99.14870971539799882, 1.872989114519528986 ) ) ;
#12216=ORIENTED_EDGE ( 'NONE', *, *, #2008, .T. ) ;
#12238=ORIENTED_EDGE ( 'NONE', *, *, #2394, .T. ) ;
#12250=PLANE ( 'NONE',  #14490 ) ;
#12269=ORIENTED_EDGE ( 'NONE', *, *, #8627, .T. ) ;
#12277=CARTESIAN_POINT ( 'NONE',  ( -8.660254037844415720, 45.00000000000001421, -4.999999999999952927 ) ) ;
#12284=CARTESIAN_POINT ( 'NONE',  ( 1.037474003217658816E-14, 92.00000000000001421, 9.080892972013893782 ) ) ;
#12296=DIRECTION ( 'NONE',  ( 0.000000000000000000, 0.000000000000000000, 1.000000000000000000 ) ) ;
#12302=LINE ( 'NONE', #2075, #2543 ) ;
#12303=CARTESIAN_POINT ( 'NONE',  ( 1.105645237078933619E-14, 82.00000000000001421, 14.08089297201389023 ) ) ;
#12330=EDGE_CURVE ( 'NONE', #9758, #3981, #8130, .T. ) ;
#12343=CARTESIAN_POINT ( 'NONE',  ( 9.574901606694759531E-15, 52.00000000000000711, -45.00000000000002842 ) ) ;
#12346=CARTESIAN_POINT ( 'NONE',  ( 0.000000000000000000, 102.0000000000000142, 5.000000000000000000 ) ) ;
#12362=CARTESIAN_POINT ( 'NONE',  ( -5.000000000000000000, 99.58041009241398456, 7.580410092413952583 ) ) ;
#12363=CARTESIAN_POINT ( 'NONE',  ( 9.227956911499398113E-15, 102.0000000000000142, -1.913737646857611713E-14 ) ) ;
#12372=VECTOR ( 'NONE', #7449, 1000.000000000000000 ) ;
#12375=CIRCLE ( 'NONE', #11063, 45.00000000000000711 ) ;
#12409=AXIS2_PLACEMENT_3D ( 'NONE', #5828, #5911, #6156 ) ;
#12433=VERTEX_POINT ( 'NONE', #2127 ) ;
#12468=ORIENTED_EDGE ( 'NONE', *, *, #4864, .T. ) ;
#12475=FACE_OUTER_BOUND ( 'NONE', #4310, .T. ) ;
#12479=DIRECTION ( 'NONE',  ( -0.3420201433256698231, 0.6644630243886754384, 0.6644630243886734400 ) ) ;
#12480=CARTESIAN_POINT ( 'NONE',  ( 5.000000000000000000, 99.58041009241404140, -7.580410092414002321 ) ) ;
#12503=DIRECTION ( 'NONE',  ( 6.938893903907231459E-18, -1.000000000000000000, -5.551115123125782702E-17 ) ) ;
#12513=EDGE_CURVE ( 'NONE', #16149, #7285, #9710, .T. ) ;
#12516=ADVANCED_FACE ( 'NONE', ( #9622 ), #6578, .T. ) ;
#12530=( BOUNDED_CURVE ( )  B_SPLINE_CURVE ( 3, ( #8951, #13922, #2539, #15340 ),
 .UNSPECIFIED., .F., .F. ) 
 B_SPLINE_CURVE_WITH_KNOTS ( ( 4, 4 ),
 ( 3.141592653589793116, 3.724683441357936609 ),
 .UNSPECIFIED. ) 
 CURVE ( )  GEOMETRIC_REPRESENTATION_ITEM ( )  RATIONAL_B_SPLINE_CURVE ( ( 1.000000000000000000, 0.9718672150731670900, 0.9718672150731670900, 1.000000000000000000 ) ) 
 REPRESENTATION_ITEM ( '' )  );
#12566=( NAMED_UNIT ( * ) PLANE_ANGLE_UNIT ( ) SI_UNIT ( $, .RADIAN. ) );
#12567=ORIENTED_EDGE ( 'NONE', *, *, #3150, .F. ) ;
#12579=CIRCLE ( 'NONE', #1144, 45.00000000000000711 ) ;
#12587=ADVANCED_FACE ( 'NONE', ( #6303 ), #10291, .T. ) ;
#12591=CIRCLE ( 'NONE', #93, 9.080892972013911546 ) ;
#12605=LINE ( 'NONE', #6545, #8079 ) ;
#12608=DIRECTION ( 'NONE',  ( -1.000000000000000000, 0.000000000000000000, 0.000000000000000000 ) ) ;
#12615=DIRECTION ( 'NONE',  ( 0.000000000000000000, 0.000000000000000000, 1.000000000000000000 ) ) ;
#12635=DIRECTION ( 'NONE',  ( 5.069245582283711292E-17, 1.000000000000000000, -8.780190904559502465E-17 ) ) ;
#12643=CARTESIAN_POINT ( 'NONE',  ( 7.580410092413973011, 99.32916037694960210, 5.000000000000000000 ) ) ;
#12653=VECTOR ( 'NONE', #5320, 1000.000000000000000 ) ;
#12657=VERTEX_POINT ( 'NONE', #9954 ) ;
#12658=CARTESIAN_POINT ( 'NONE',  ( 5.000000000000000000, 94.44606029984966256, 0.2275664557063671878 ) ) ;
#12708=ORIENTED_EDGE ( 'NONE', *, *, #8637, .T. ) ;
#12720=CARTESIAN_POINT ( 'NONE',  ( -7.580410092413979228, 101.3368000520362813, -5.000000000000000000 ) ) ;
#12729=VERTEX_POINT ( 'NONE', #4044 ) ;
#12752=EDGE_LOOP ( 'NONE', ( #5084, #700 ) ) ;
#12775=CARTESIAN_POINT ( 'NONE',  ( 5.288637809679021457E-15, 52.00000000000001421, -35.00000000000002842 ) ) ;
#12783=DIRECTION ( 'NONE',  ( -6.938893903907231459E-18, 1.000000000000000000, 5.551115123125782702E-17 ) ) ;
#12784=VERTEX_POINT ( 'NONE', #456 ) ;
#12787=CARTESIAN_POINT ( 'NONE',  ( 7.580410092413973011, 101.3368000520362813, 5.000000000000000000 ) ) ;
#12796=CARTESIAN_POINT ( 'NONE',  ( 1.790468199911986025, 98.25246584726779986, -9.080892972013931086 ) ) ;
#12808=CARTESIAN_POINT ( 'NONE',  ( 5.000000000000000000, 90.58578643762692195, 1.414213562373097588 ) ) ;
#12809=EDGE_CURVE ( 'NONE', #5951, #12657, #1459, .T. ) ;
#12828=VECTOR ( 'NONE', #12065, 1000.000000000000114 ) ;
#12839=EDGE_CURVE ( 'NONE', #8062, #332, #11902, .T. ) ;
#12841=FACE_OUTER_BOUND ( 'NONE', #10537, .T. ) ;
#12857=DIRECTION ( 'NONE',  ( 0.000000000000000000, 0.000000000000000000, -1.000000000000000000 ) ) ;
#12860=DIRECTION ( 'NONE',  ( -1.000000000000000000, 0.000000000000000000, -0.000000000000000000 ) ) ;
#12865=CARTESIAN_POINT ( 'NONE',  ( 9.574901606694759531E-15, 52.00000000000001421, -2.191293403013901163E-14 ) ) ;
#12874=EDGE_CURVE ( 'NONE', #14188, #3621, #10365, .T. ) ;
#12885=CARTESIAN_POINT ( 'NONE',  ( 1.790468199911983804, 98.25246584726775723, 9.080892972013892006 ) ) ;
#12902=MECHANICAL_DESIGN_GEOMETRIC_PRESENTATION_REPRESENTATION('',(#6543),#4676);
#12947=CARTESIAN_POINT ( 'NONE',  ( 5.000000000000000000, 99.58041009241404140, -7.580410092414002321 ) ) ;
#12950=LINE ( 'NONE', #2328, #12653 ) ;
#12963=PLANE ( 'NONE',  #7049 ) ;
#12964=CARTESIAN_POINT ( 'NONE',  ( 5.000000000000000888, 91.24478243472064776, -8.497612305159609747 ) ) ;
#13040=ORIENTED_EDGE ( 'NONE', *, *, #2345, .F. ) ;
#13053=CARTESIAN_POINT ( 'NONE',  ( 5.000000000000000000, 96.75198296766781425, 7.580410092413965017 ) ) ;
#13065=LINE ( 'NONE', #6766, #5747 ) ;
#13083=CARTESIAN_POINT ( 'NONE',  ( -7.580410092413979228, 99.32916037694960210, -5.000000000000000000 ) ) ;
#13115=ORIENTED_EDGE ( 'NONE', *, *, #8637, .F. ) ;
#13135=ORIENTED_EDGE ( 'NONE', *, *, #1, .T. ) ;
#13141=LINE ( 'NONE', #10582, #7608 ) ;
#13191=DIRECTION ( 'NONE',  ( 6.938893903907231459E-18, -1.000000000000000000, -5.551115123125782702E-17 ) ) ;
#13203=DIRECTION ( 'NONE',  ( -0.000000000000000000, -0.7071067811865487940, -0.7071067811865463515 ) ) ;
#13245=CARTESIAN_POINT ( 'NONE',  ( -7.581784256837357461, 125.2766624725656897, 36.10508959731173917 ) ) ;
#13257=( BOUNDED_CURVE ( )  B_SPLINE_CURVE ( 3, ( #9069, #12885, #15374, #13053 ),
 .UNSPECIFIED., .F., .T. ) 
 B_SPLINE_CURVE_WITH_KNOTS ( ( 4, 4 ),
 ( 3.141592653589793116, 3.724683441357936609 ),
 .UNSPECIFIED. ) 
 CURVE ( )  GEOMETRIC_REPRESENTATION_ITEM ( )  RATIONAL_B_SPLINE_CURVE ( ( 1.000000000000000000, 0.9718672150731670900, 0.9718672150731670900, 1.000000000000000000 ) ) 
 REPRESENTATION_ITEM ( '' )  );
#13258=EDGE_LOOP ( 'NONE', ( #5660, #16104, #14777, #3722 ) ) ;
#13288=CARTESIAN_POINT ( 'NONE',  ( 0.000000000000000000, 102.0000000000000142, -5.000000000000000000 ) ) ;
#13316=EDGE_CURVE ( 'NONE', #6916, #306, #13141, .T. ) ;
#13371=ORIENTED_EDGE ( 'NONE', *, *, #10222, .T. ) ;
#13378=DIRECTION ( 'NONE',  ( 0.000000000000000000, 0.000000000000000000, -1.000000000000000000 ) ) ;
#13394=DIRECTION ( 'NONE',  ( 0.1984322509960772252, -0.9259215214979057418, -0.3213938048432687378 ) ) ;
#13396=CARTESIAN_POINT ( 'NONE',  ( -2.020067798342124465, 103.3979712344554116, 5.000000000000000000 ) ) ;
#13398=CARTESIAN_POINT ( 'NONE',  ( 1.508581220285784909E-14, 52.00000000000002132, 44.99999999999998579 ) ) ;
#13427=DIRECTION ( 'NONE',  ( -0.9961946980917455452, -0.08715574274765824914, 0.000000000000000000 ) ) ;
#13441=EDGE_CURVE ( 'NONE', #3153, #3704, #13065, .T. ) ;
#13511=EDGE_CURVE ( 'NONE', #12729, #12156, #12302, .T. ) ;
#13530=CARTESIAN_POINT ( 'NONE',  ( 9.574901606694759531E-15, 52.00000000000001421, -2.191293403013901479E-14 ) ) ;
#13534=FACE_OUTER_BOUND ( 'NONE', #15613, .T. ) ;
#13555=DIRECTION ( 'NONE',  ( 0.000000000000000000, -5.551115123125782702E-17, 1.000000000000000000 ) ) ;
#13574=DIRECTION ( 'NONE',  ( 0.3420201433256697676, 0.6644630243886755494, -0.6644630243886733290 ) ) ;
#13578=ORIENTED_EDGE ( 'NONE', *, *, #8336, .F. ) ;
#13593=VERTEX_POINT ( 'NONE', #15119 ) ;
#13599=ORIENTED_EDGE ( 'NONE', *, *, #2775, .T. ) ;
#13602=DIRECTION ( 'NONE',  ( 6.938893903907231459E-18, -1.000000000000000000, -5.551115123125782702E-17 ) ) ;
#13604=DIRECTION ( 'NONE',  ( -0.3213938048432674610, 0.7471788047720969717, 0.5817472440052537941 ) ) ;
#13609=DIRECTION ( 'NONE',  ( 0.000000000000000000, 0.000000000000000000, -1.000000000000000000 ) ) ;
#13626=CARTESIAN_POINT ( 'NONE',  ( -7.580410092413954359, 102.0000000000000142, 5.000000000000000000 ) ) ;
#13660=AXIS2_PLACEMENT_3D ( 'NONE', #8658, #16227, #14635 ) ;
#13702=CIRCLE ( 'NONE', #9200, 14.08089297201391155 ) ;
#13711=CARTESIAN_POINT ( 'NONE',  ( 9.227956911499398113E-15, 102.0000000000000142, -1.913737646857611713E-14 ) ) ;
#13722=VECTOR ( 'NONE', #15937, 1000.000000000000000 ) ;
#13729=EDGE_LOOP ( 'NONE', ( #16170, #5205, #1802, #3196 ) ) ;
#13739=CARTESIAN_POINT ( 'NONE',  ( 7.580410092413973011, 99.32916037694960210, 5.000000000000000000 ) ) ;
#13780=DIRECTION ( 'NONE',  ( 0.3420201433256697121, -0.6644630243886754384, -0.6644630243886734400 ) ) ;
#13792=CARTESIAN_POINT ( 'NONE',  ( -5.000000000000000000, 100.8332763660826572, -11.66170349082880442 ) ) ;
#13799=ADVANCED_FACE ( 'NONE', ( #4246, #9312 ), #14365, .T. ) ;
#13854=DIRECTION ( 'NONE',  ( 6.938893903907231459E-18, -1.000000000000000000, -5.551115123125782702E-17 ) ) ;
#13862=ORIENTED_EDGE ( 'NONE', *, *, #2345, .T. ) ;
#13863=ORIENTED_EDGE ( 'NONE', *, *, #2842, .T. ) ;
#13869=CARTESIAN_POINT ( 'NONE',  ( 9.574901606694759531E-15, 52.00000000000001421, -2.191293403013901479E-14 ) ) ;
#13887=LINE ( 'NONE', #6684, #3343 ) ;
#13922=CARTESIAN_POINT ( 'NONE',  ( 1.790468199911983804, 101.0808929720139275, 9.080892972013892006 ) ) ;
#13928=CIRCLE ( 'NONE', #6512, 24.08089297201390977 ) ;
#13955=VECTOR ( 'NONE', #6998, 1000.000000000000114 ) ;
#13972=ORIENTED_EDGE ( 'NONE', *, *, #7282, .F. ) ;
#13978=VECTOR ( 'NONE', #12503, 1000.000000000000000 ) ;
#14015=EDGE_CURVE ( 'NONE', #10751, #12784, #5981, .T. ) ;
#14023=ADVANCED_FACE ( 'NONE', ( #8245 ), #14705, .F. ) ;
#14024=LINE ( 'NONE', #8966, #14392 ) ;
#14073=ORIENTED_EDGE ( 'NONE', *, *, #9514, .F. ) ;
#14110=CARTESIAN_POINT ( 'NONE',  ( 14.43699227201001101, 100.7369268407877598, -5.000000000000000000 ) ) ;
#14118=FACE_OUTER_BOUND ( 'NONE', #7156, .T. ) ;
#14129=FILL_AREA_STYLE_COLOUR ( '', #6795 ) ;
#14173=DIRECTION ( 'NONE',  ( -6.938893903907231459E-18, 1.000000000000000000, 5.551115123125782702E-17 ) ) ;
#14175=DIRECTION ( 'NONE',  ( 0.9361168066628590134, -0.08189960831908912886, 0.3420201433256691570 ) ) ;
#14180=VECTOR ( 'NONE', #6786, 1000.000000000000114 ) ;
#14188=VERTEX_POINT ( 'NONE', #14205 ) ;
#14205=CARTESIAN_POINT ( 'NONE',  ( -5.000000000000000000, 99.58041009241402719, -7.580410092413988998 ) ) ;
#14208=ORIENTED_EDGE ( 'NONE', *, *, #6165, .F. ) ;
#14229=CIRCLE ( 'NONE', #953, 14.08089297201391155 ) ;
#14250=DIRECTION ( 'NONE',  ( 0.000000000000000000, 0.7071067811865487940, -0.7071067811865463515 ) ) ;
#14274=ADVANCED_FACE ( 'NONE', ( #8058 ), #6498, .F. ) ;
#14276=DIRECTION ( 'NONE',  ( 0.000000000000000000, 0.000000000000000000, -1.000000000000000000 ) ) ;
#14277=ORIENTED_EDGE ( 'NONE', *, *, #8336, .T. ) ;
#14295=ORIENTED_EDGE ( 'NONE', *, *, #11199, .F. ) ;
#14308=EDGE_CURVE ( 'NONE', #2312, #10814, #14529, .T. ) ;
#14312=CARTESIAN_POINT ( 'NONE',  ( 7.580410092413998768, 101.3368000520362813, -5.000000000000000000 ) ) ;
#14349=PRODUCT_CONTEXT ( 'NONE', #2269, 'mechanical' ) ;
#14356=ORIENTED_EDGE ( 'NONE', *, *, #9936, .F. ) ;
#14365=PLANE ( 'NONE',  #2289 ) ;
#14369=LINE ( 'NONE', #321, #16399 ) ;
#14373=EDGE_LOOP ( 'NONE', ( #8630, #2167, #5629, #14889 ) ) ;
#14392=VECTOR ( 'NONE', #5328, 1000.000000000000000 ) ;
#14408=CARTESIAN_POINT ( 'NONE',  ( 4.350898428888834396E-14, 37.00000000000001421, 10.00000000000000355 ) ) ;
#14413=CARTESIAN_POINT ( 'NONE',  ( -9.642970592016627762, 99.14870971539799882, -1.872989114519522547 ) ) ;
#14422=VECTOR ( 'NONE', #1890, 1000.000000000000114 ) ;
#14454=CARTESIAN_POINT ( 'NONE',  ( -8.660254037844415720, 37.00000000000001421, -4.999999999999952038 ) ) ;
#14488=ORIENTED_EDGE ( 'NONE', *, *, #4528, .T. ) ;
#14490=AXIS2_PLACEMENT_3D ( 'NONE', #686, #5861, #853 ) ;
#14506=CONICAL_SURFACE ( 'NONE', #698, 35.00000000000000711, 0.3490658503988666728 ) ;
#14526=DIRECTION ( 'NONE',  ( 0.000000000000000000, 0.000000000000000000, 1.000000000000000000 ) ) ;
#14529=LINE ( 'NONE', #5656, #6719 ) ;
#14537=CARTESIAN_POINT ( 'NONE',  ( 9.220054415934899174E-15, 45.00000000000001421, -2.129832066681984848E-14 ) ) ;
#14545=EDGE_CURVE ( 'NONE', #1879, #3153, #4913, .T. ) ;
#14563=DIRECTION ( 'NONE',  ( 0.000000000000000000, 0.000000000000000000, 1.000000000000000000 ) ) ;
#14572=ORIENTED_EDGE ( 'NONE', *, *, #2049, .T. ) ;
#14574=ORIENTED_EDGE ( 'NONE', *, *, #10387, .T. ) ;
#14581=CARTESIAN_POINT ( 'NONE',  ( -5.000000000000000000, 96.75198296766782846, -7.580410092413988998 ) ) ;
#14621=CARTESIAN_POINT ( 'NONE',  ( 9.220054415934899174E-15, 45.00000000000001421, -2.129832066681984848E-14 ) ) ;
#14628=EDGE_CURVE ( 'NONE', #306, #15764, #14024, .T. ) ;
#14635=DIRECTION ( 'NONE',  ( 0.000000000000000000, 0.000000000000000000, 1.000000000000000000 ) ) ;
#14649=EDGE_CURVE ( 'NONE', #1407, #15190, #6192, .T. ) ;
#14652=ORIENTED_EDGE ( 'NONE', *, *, #14933, .T. ) ;
#14653=EDGE_CURVE ( 'NONE', #11207, #8062, #2639, .T. ) ;
#14660=CARTESIAN_POINT ( 'NONE',  ( 9.253960653386475815E-15, 98.25246584726779986, -9.080892972013931086 ) ) ;
#14681=VECTOR ( 'NONE', #12479, 1000.000000000000114 ) ;
#14683=CYLINDRICAL_SURFACE ( 'NONE', #1690, 9.080892972013911546 ) ;
#14697=ORIENTED_EDGE ( 'NONE', *, *, #7178, .T. ) ;
#14705=PLANE ( 'NONE',  #7874 ) ;
#14724=CARTESIAN_POINT ( 'NONE',  ( 9.642970592016636644, 99.14870971539799882, 1.872989114519530984 ) ) ;
#14737=ORIENTED_EDGE ( 'NONE', *, *, #14649, .F. ) ;
#14752=AXIS2_PLACEMENT_3D ( 'NONE', #16065, #5940, #4697 ) ;
#14755=AXIS2_PLACEMENT_3D ( 'NONE', #6177, #4944, #14972 ) ;
#14761=DIRECTION ( 'NONE',  ( 0.000000000000000000, 0.000000000000000000, 1.000000000000000000 ) ) ;
#14768=LINE ( 'NONE', #11044, #9815 ) ;
#14771=CARTESIAN_POINT ( 'NONE',  ( 9.297345850538470396E-15, 92.00000000000001421, -14.08089297201393109 ) ) ;
#14777=ORIENTED_EDGE ( 'NONE', *, *, #3607, .F. ) ;
#14778=VERTEX_POINT ( 'NONE', #3294 ) ;
#14785=DIRECTION ( 'NONE',  ( 0.3420201433256697676, -0.6644630243886755494, -0.6644630243886733290 ) ) ;
#14791=FACE_BOUND ( 'NONE', #6989, .T. ) ;
#14795=LINE ( 'NONE', #5761, #3120 ) ;
#14800=ORIENTED_EDGE ( 'NONE', *, *, #15871, .T. ) ;
#14835=CIRCLE ( 'NONE', #16182, 9.080892972013911546 ) ;
#14863=ORIENTED_EDGE ( 'NONE', *, *, #14653, .F. ) ;
#14877=CARTESIAN_POINT ( 'NONE',  ( 5.000000000000000000, 0.000000000000000000, 0.000000000000000000 ) ) ;
#14889=ORIENTED_EDGE ( 'NONE', *, *, #14545, .F. ) ;
#14901=PLANE ( 'NONE',  #10787 ) ;
#14910=LINE ( 'NONE', #12343, #11047 ) ;
#14933=EDGE_CURVE ( 'NONE', #15902, #15466, #4978, .T. ) ;
#14938=CIRCLE ( 'NONE', #6747, 10.00000000000000355 ) ;
#14945=ORIENTED_EDGE ( 'NONE', *, *, #10387, .F. ) ;
#14953=CARTESIAN_POINT ( 'NONE',  ( 9.297345850538470396E-15, 92.00000000000001421, -1.969248798088869855E-14 ) ) ;
#14957=CARTESIAN_POINT ( 'NONE',  ( 5.000000000000000000, 96.75198296766784267, -7.580410092414001433 ) ) ;
#14970=LINE ( 'NONE', #12157, #3859 ) ;
#14972=DIRECTION ( 'NONE',  ( 0.000000000000000000, 0.000000000000000000, 1.000000000000000000 ) ) ;
#15011=CARTESIAN_POINT ( 'NONE',  ( -5.000000000000000000, 121.6750890729883565, 29.67508907298824283 ) ) ;
#15020=AXIS2_PLACEMENT_3D ( 'NONE', #7995, #8073, #1755 ) ;
#15037=ORIENTED_EDGE ( 'NONE', *, *, #1049, .F. ) ;
#15038=PLANE ( 'NONE',  #8885 ) ;
#15043=CYLINDRICAL_SURFACE ( 'NONE', #492, 10.00000000000000355 ) ;
#15044=CARTESIAN_POINT ( 'NONE',  ( -5.000000000000000000, 90.58578643762692195, 1.414213562373097588 ) ) ;
#15057=SURFACE_SIDE_STYLE ('',( #7820 ) ) ;
#15097=CARTESIAN_POINT ( 'NONE',  ( -5.000000000000000000, 0.000000000000000000, 0.000000000000000000 ) ) ;
#15119=CARTESIAN_POINT ( 'NONE',  ( 9.397478011314830142E-15, 52.00000000000000711, -45.00000000000002842 ) ) ;
#15122=FACE_OUTER_BOUND ( 'NONE', #11461, .T. ) ;
#15140=CARTESIAN_POINT ( 'NONE',  ( 9.297345850538470396E-15, 92.00000000000001421, -1.969248798088869855E-14 ) ) ;
#15171=DIRECTION ( 'NONE',  ( 0.9961946980917455452, 0.08715574274765824914, 0.000000000000000000 ) ) ;
#15181=LINE ( 'NONE', #3812, #11629 ) ;
#15190=VERTEX_POINT ( 'NONE', #9660 ) ;
#15196=CARTESIAN_POINT ( 'NONE',  ( -8.660254037844415720, 37.00000000000001421, -4.999999999999952038 ) ) ;
#15205=ORIENTED_EDGE ( 'NONE', *, *, #6318, .T. ) ;
#15209=( LENGTH_UNIT ( ) NAMED_UNIT ( * ) SI_UNIT ( .MILLI., .METRE. ) );
#15215=DIRECTION ( 'NONE',  ( 0.9361168066628590134, -0.08189960831908912886, 0.3420201433256691570 ) ) ;
#15230=VERTEX_POINT ( 'NONE', #7098 ) ;
#15238=EDGE_CURVE ( 'NONE', #3904, #9419, #6012, .T. ) ;
#15251=CARTESIAN_POINT ( 'NONE',  ( -1.790468199911976477, 98.25246584726777144, 9.080892972013895559 ) ) ;
#15253=ORIENTED_EDGE ( 'NONE', *, *, #10491, .T. ) ;
#15256=STYLED_ITEM ( 'NONE', ( #1330 ), #8709 ) ;
#15276=DIRECTION ( 'NONE',  ( -0.000000000000000000, 0.7890408728378112135, -0.6143407043256575717 ) ) ;
#15303=ORIENTED_EDGE ( 'NONE', *, *, #5021, .T. ) ;
#15314=CIRCLE ( 'NONE', #9754, 9.080892972013911546 ) ;
#15340=CARTESIAN_POINT ( 'NONE',  ( 5.000000000000000000, 99.58041009241399877, 7.580410092413963241 ) ) ;
#15354=CIRCLE ( 'NONE', #2879, 45.00000000000000711 ) ;
#15361=PLANE ( 'NONE',  #6284 ) ;
#15372=DIRECTION ( 'NONE',  ( 5.069245582283711292E-17, 1.000000000000000000, -8.780190904559502465E-17 ) ) ;
#15374=CARTESIAN_POINT ( 'NONE',  ( 3.505380114644273348, 97.73782665365219202, 8.566253778398346341 ) ) ;
#15376=CARTESIAN_POINT ( 'NONE',  ( 0.000000000000000000, 0.000000000000000000, 5.000000000000000000 ) ) ;
#15398=LINE ( 'NONE', #182, #13978 ) ;
#15420=LINE ( 'NONE', #6636, #11013 ) ;
#15425=FACE_BOUND ( 'NONE', #12752, .T. ) ;
#15450=DIRECTION ( 'NONE',  ( 0.000000000000000000, 0.000000000000000000, 1.000000000000000000 ) ) ;
#15466=VERTEX_POINT ( 'NONE', #4343 ) ;
#15468=DIRECTION ( 'NONE',  ( -6.938893903907231459E-18, 1.000000000000000000, 5.551115123125782702E-17 ) ) ;
#15494=ADVANCED_FACE ( 'NONE', ( #499 ), #5359, .F. ) ;
#15499=DIRECTION ( 'NONE',  ( 5.069245582283711292E-17, 1.000000000000000000, -8.780190904559503697E-17 ) ) ;
#15504=CARTESIAN_POINT ( 'NONE',  ( 9.366734789577542680E-15, 82.00000000000001421, -2.024759949320127682E-14 ) ) ;
#15519=ORIENTED_EDGE ( 'NONE', *, *, #8241, .F. ) ;
#15530=LINE ( 'NONE', #1888, #16433 ) ;
#15537=VECTOR ( 'NONE', #11636, 1000.000000000000114 ) ;
#15556=EDGE_CURVE ( 'NONE', #798, #1879, #5669, .T. ) ;
#15557=DIRECTION ( 'NONE',  ( 0.000000000000000000, 0.000000000000000000, 1.000000000000000000 ) ) ;
#15558=VECTOR ( 'NONE', #14250, 1000.000000000000000 ) ;
#15566=CIRCLE ( 'NONE', #2288, 10.00000000000000355 ) ;
#15567=VECTOR ( 'NONE', #6641, 1000.000000000000000 ) ;
#15606=CARTESIAN_POINT ( 'NONE',  ( 3.465800365507340608, 94.69943522268255265, -5.000000000000000000 ) ) ;
#15609=ORIENTED_EDGE ( 'NONE', *, *, #8123, .F. ) ;
#15613=EDGE_LOOP ( 'NONE', ( #1915, #7033, #4043, #9113, #4149, #15783, #11283, #10851, #10446, #3958, #13371, #7883 ) ) ;
#15637=ORIENTED_EDGE ( 'NONE', *, *, #6628, .T. ) ;
#15661=EDGE_CURVE ( 'NONE', #9035, #8437, #14938, .T. ) ;
#15665=DIRECTION ( 'NONE',  ( 6.938893903907231459E-18, -1.000000000000000000, -5.551115123125782702E-17 ) ) ;
#15681=DIRECTION ( 'NONE',  ( 6.938893903907231459E-18, -1.000000000000000000, -5.551115123125782702E-17 ) ) ;
#15696=SHAPE_REPRESENTATION_RELATIONSHIP ( 'NONE' , 'NONE' ,  #10113, #8007 ) ;
#15705=ORIENTED_EDGE ( 'NONE', *, *, #13511, .F. ) ;
#15708=DIRECTION ( 'NONE',  ( 0.000000000000000000, 1.541976423090494894E-16, 1.000000000000000000 ) ) ;
#15754=LINE ( 'NONE', #3041, #7301 ) ;
#15764=VERTEX_POINT ( 'NONE', #4584 ) ;
#15778=SURFACE_SIDE_STYLE ('',( #10717 ) ) ;
#15781=DIRECTION ( 'NONE',  ( -0.000000000000000000, -0.7071067811865487940, -0.7071067811865463515 ) ) ;
#15783=ORIENTED_EDGE ( 'NONE', *, *, #5622, .F. ) ;
#15803=CARTESIAN_POINT ( 'NONE',  ( -1.790468199911972924, 101.0808929720139702, -9.080892972013931086 ) ) ;
#15812=AXIS2_PLACEMENT_3D ( 'NONE', #2158, #11073, #8560 ) ;
#15813=DIRECTION ( 'NONE',  ( -0.9777979793268667397, -0.2095497831645171394, -0.000000000000000000 ) ) ;
#15822=CARTESIAN_POINT ( 'NONE',  ( -21.98588717320197006, 102.5902090043563533, -5.000000000000000000 ) ) ;
#15863=DIRECTION ( 'NONE',  ( -6.938893903907231459E-18, 1.000000000000000000, 5.551115123125782702E-17 ) ) ;
#15866=CARTESIAN_POINT ( 'NONE',  ( -14.43699227201014423, 100.7369268407877456, 5.000000000000000000 ) ) ;
#15871=EDGE_CURVE ( 'NONE', #1602, #16014, #7150, .T. ) ;
#15875=ORIENTED_EDGE ( 'NONE', *, *, #7282, .T. ) ;
#15894=CARTESIAN_POINT ( 'NONE',  ( -41.80721665588497160, 98.34234248903787545, -5.000000000000000000 ) ) ;
#15902=VERTEX_POINT ( 'NONE', #13792 ) ;
#15937=DIRECTION ( 'NONE',  ( 6.938893903907231459E-18, -1.000000000000000000, -5.551115123125782702E-17 ) ) ;
#15939=CARTESIAN_POINT ( 'NONE',  ( 4.391452393547104422E-14, 45.00000000000001421, 10.00000000000000355 ) ) ;
#15947=EDGE_CURVE ( 'NONE', #10158, #11932, #8807, .T. ) ;
#15980=DIRECTION ( 'NONE',  ( -5.069245582283711292E-17, -1.000000000000000000, 8.780190904559502465E-17 ) ) ;
#15988=PLANE ( 'NONE',  #8935 ) ;
#16013=ORIENTED_EDGE ( 'NONE', *, *, #12809, .T. ) ;
#16014=VERTEX_POINT ( 'NONE', #11235 ) ;
#16016=CARTESIAN_POINT ( 'NONE',  ( 9.574901606694759531E-15, 52.00000000000001421, -2.191293403013901163E-14 ) ) ;
#16020=CARTESIAN_POINT ( 'NONE',  ( 5.000000000000000000, 100.8332763660827567, 11.66170349082890212 ) ) ;
#16025=LINE ( 'NONE', #14771, #6776 ) ;
#16029=EDGE_LOOP ( 'NONE', ( #1103, #4777 ) ) ;
#16056=ORIENTED_EDGE ( 'NONE', *, *, #10694, .T. ) ;
#16061=MECHANICAL_DESIGN_GEOMETRIC_PRESENTATION_REPRESENTATION('',(#15256),#642);
#16065=CARTESIAN_POINT ( 'NONE',  ( 9.366734789577542680E-15, 82.00000000000001421, -2.024759949320127682E-14 ) ) ;
#16078=VERTEX_POINT ( 'NONE', #235 ) ;
#16083=VECTOR ( 'NONE', #537, 1000.000000000000114 ) ;
#16085=VECTOR ( 'NONE', #15468, 1000.000000000000000 ) ;
#16104=ORIENTED_EDGE ( 'NONE', *, *, #15556, .T. ) ;
#16126=EDGE_LOOP ( 'NONE', ( #9131, #3903 ) ) ;
#16130=( BOUNDED_CURVE ( )  B_SPLINE_CURVE ( 3, ( #5675, #15803, #10504, #7918 ),
 .UNSPECIFIED., .F., .T. ) 
 B_SPLINE_CURVE_WITH_KNOTS ( ( 4, 4 ),
 ( 3.141592653589793116, 3.724683441357938829 ),
 .UNSPECIFIED. ) 
 CURVE ( )  GEOMETRIC_REPRESENTATION_ITEM ( )  RATIONAL_B_SPLINE_CURVE ( ( 1.000000000000000000, 0.9718672150731668680, 0.9718672150731668680, 1.000000000000000000 ) ) 
 REPRESENTATION_ITEM ( '' )  );
#16149=VERTEX_POINT ( 'NONE', #4244 ) ;
#16166=EDGE_CURVE ( 'NONE', #5951, #13593, #12579, .T. ) ;
#16170=ORIENTED_EDGE ( 'NONE', *, *, #10694, .F. ) ;
#16182=AXIS2_PLACEMENT_3D ( 'NONE', #2384, #7710, #12615 ) ;
#16201=DIRECTION ( 'NONE',  ( 0.000000000000000000, -0.6143407043256605693, 0.7890408728378088821 ) ) ;
#16208=PLANE ( 'NONE',  #12409 ) ;
#16210=ORIENTED_EDGE ( 'NONE', *, *, #8343, .T. ) ;
#16226=VERTEX_POINT ( 'NONE', #15866 ) ;
#16227=DIRECTION ( 'NONE',  ( -6.938893903907231459E-18, 1.000000000000000000, 5.551115123125782702E-17 ) ) ;
#16237=CARTESIAN_POINT ( 'NONE',  ( 7.580410092413998768, 99.32916037694960210, -5.000000000000000000 ) ) ;
#16239=CARTESIAN_POINT ( 'NONE',  ( -8.487905985326110070, 94.05711243240941144, -4.885539557155581747 ) ) ;
#16251=CARTESIAN_POINT ( 'NONE',  ( 7.580410092413998768, 101.3368000520362813, -5.000000000000000000 ) ) ;
#16277=ORIENTED_EDGE ( 'NONE', *, *, #12839, .F. ) ;
#16281=VERTEX_POINT ( 'NONE', #5600 ) ;
#16344=ORIENTED_EDGE ( 'NONE', *, *, #8539, .T. ) ;
#16346=PRODUCT_DEFINITION_FORMATION_WITH_SPECIFIED_SOURCE ( 'ANY', '', #6681, .NOT_KNOWN. ) ;
#16348=DIRECTION ( 'NONE',  ( -3.536495997885206014E-17, -0.9396926207859082059, -0.3420201433256695456 ) ) ;
#16351=VECTOR ( 'NONE', #5457, 1000.000000000000227 ) ;
#16372=CARTESIAN_POINT ( 'NONE',  ( 14.26268078651494342, 98.74453744460424787, -5.000000000000000000 ) ) ;
#16376=DIRECTION ( 'NONE',  ( -6.938893903907231459E-18, 1.000000000000000000, 5.551115123125782702E-17 ) ) ;
#16394=DIRECTION ( 'NONE',  ( 0.000000000000000000, -0.7071067811865487940, -0.7071067811865463515 ) ) ;
#16399=VECTOR ( 'NONE', #3151, 1000.000000000000000 ) ;
#16402=ADVANCED_FACE ( 'NONE', ( #9827 ), #4514, .F. ) ;
#16407=DIRECTION ( 'NONE',  ( 6.938893903907231459E-18, -1.000000000000000000, -5.551115123125782702E-17 ) ) ;
#16415=ORIENTED_EDGE ( 'NONE', *, *, #14653, .T. ) ;
#16433=VECTOR ( 'NONE', #477, 1000.000000000000227 ) ;
#16439=DIRECTION ( 'NONE',  ( -6.938893903907231459E-18, 1.000000000000000000, 5.551115123125782702E-17 ) ) ;
ENDSEC;
END-ISO-10303-21;
